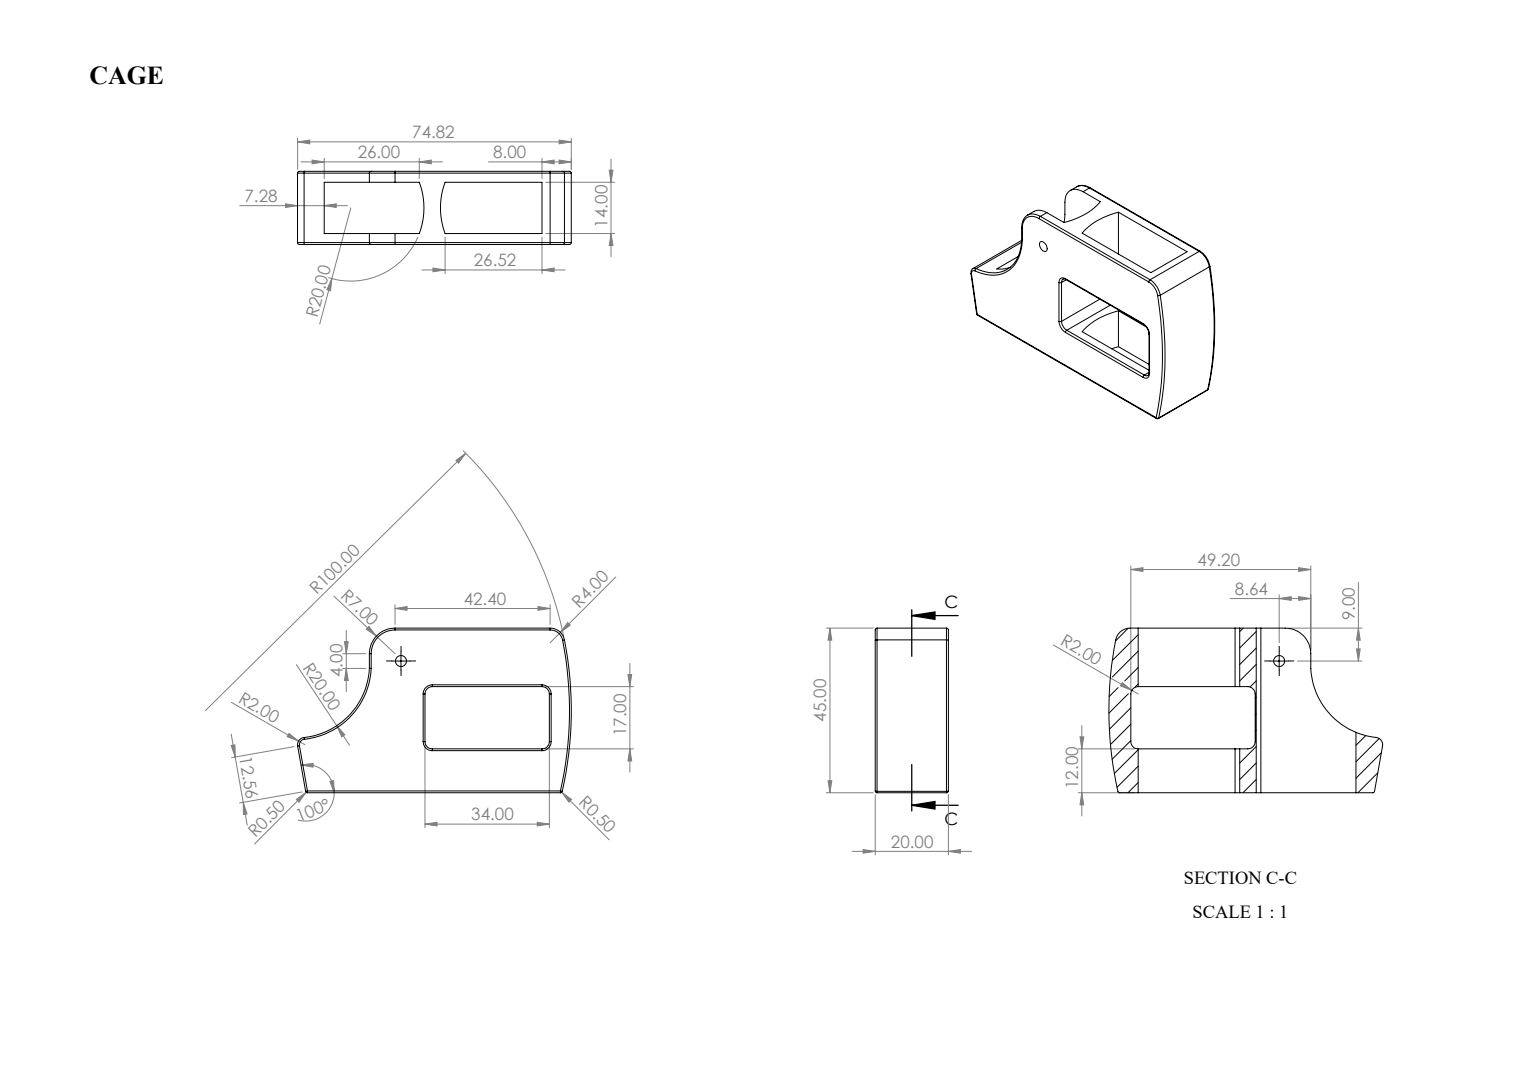
ISO-10303-21;
HEADER;
FILE_DESCRIPTION (('STEP AP214'),
    '1' );
FILE_NAME ('1.1 Cage.step',
    '2026-10-07T05:30:18',
    ( '' ),
    ( '' ),
    'SwSTEP 2.0',
    'SolidWorks 2021',
    '' );
FILE_SCHEMA (( 'AUTOMOTIVE_DESIGN' ));
ENDSEC;

DATA;
#41=DIRECTION ( 'NONE',  ( 1.000000000000000000, -5.818595309480553908E-17, 0.000000000000000000 ) ) ;
#61=ORIENTED_EDGE ( 'NONE', *, *, #8376, .F. ) ;
#102=DIRECTION ( 'NONE',  ( 0.000000000000000000, 0.000000000000000000, 1.000000000000000000 ) ) ;
#168=EDGE_LOOP ( 'NONE', ( #11039, #37677, #32498, #88509 ) ) ;
#188=DIRECTION ( 'NONE',  ( 0.000000000000000000, 0.000000000000000000, -1.000000000000000000 ) ) ;
#215=VECTOR ( 'NONE', #1501, 1000.000000000000000 ) ;
#223=DIRECTION ( 'NONE',  ( -1.000000000000000000, 0.000000000000000000, 0.000000000000000000 ) ) ;
#244=CARTESIAN_POINT ( 'NONE',  ( 17.35999999999999943, 37.99999999999997868, -7.000000000000000888 ) ) ;
#295=VERTEX_POINT ( 'NONE', #12397 ) ;
#330=ORIENTED_EDGE ( 'NONE', *, *, #68148, .F. ) ;
#338=ADVANCED_FACE ( 'NONE', ( #83350 ), #59848, .T. ) ;
#341=ORIENTED_EDGE ( 'NONE', *, *, #63443, .F. ) ;
#348=EDGE_CURVE ( 'NONE', #78868, #92229, #98382, .T. ) ;
#354=CYLINDRICAL_SURFACE ( 'NONE', #94314, 1.500000000000001332 ) ;
#363=( NAMED_UNIT ( * ) PLANE_ANGLE_UNIT ( ) SI_UNIT ( $, .RADIAN. ) );
#376=DIRECTION ( 'NONE',  ( 8.673617379884028570E-16, 1.000000000000000000, 0.000000000000000000 ) ) ;
#416=EDGE_CURVE ( 'NONE', #77981, #78868, #23450, .T. ) ;
#435=CIRCLE ( 'NONE', #56286, 0.5000000000000004441 ) ;
#442=VECTOR ( 'NONE', #21341, 1000.000000000000000 ) ;
#515=AXIS2_PLACEMENT_3D ( 'NONE', #48897, #3417, #2454 ) ;
#622=ORIENTED_EDGE ( 'NONE', *, *, #68148, .T. ) ;
#624=EDGE_CURVE ( 'NONE', #55254, #84180, #16333, .T. ) ;
#646=CIRCLE ( 'NONE', #50126, 0.5000000000000004441 ) ;
#683=EDGE_LOOP ( 'NONE', ( #89286, #70772, #2079, #80343 ) ) ;
#743=DIRECTION ( 'NONE',  ( 0.000000000000000000, 1.000000000000000000, 0.000000000000000000 ) ) ;
#779=ORIENTED_EDGE ( 'NONE', *, *, #18509, .T. ) ;
#805=ORIENTED_EDGE ( 'NONE', *, *, #45534, .F. ) ;
#821=DIRECTION ( 'NONE',  ( 1.000000000000000000, 0.000000000000000000, 5.329070518200751394E-15 ) ) ;
#842=PRODUCT_DEFINITION_FORMATION_WITH_SPECIFIED_SOURCE ( 'ANY', '', #6128, .NOT_KNOWN. ) ;
#860=DIRECTION ( 'NONE',  ( -1.000000000000000000, 0.000000000000000000, 0.000000000000000000 ) ) ;
#985=CARTESIAN_POINT ( 'NONE',  ( 32.06412365047463453, 14.00000000000001066, 9.500000000000000000 ) ) ;
#1075=VECTOR ( 'NONE', #35109, 1000.000000000000000 ) ;
#1105=LINE ( 'NONE', #77561, #75163 ) ;
#1127=DIRECTION ( 'NONE',  ( -0.000000000000000000, -0.000000000000000000, -1.000000000000000000 ) ) ;
#1194=VERTEX_POINT ( 'NONE', #53106 ) ;
#1221=CIRCLE ( 'NONE', #85851, 2.500000000000002220 ) ;
#1239=DIRECTION ( 'NONE',  ( -1.000000000000000000, 0.000000000000000000, -0.000000000000000000 ) ) ;
#1268=EDGE_CURVE ( 'NONE', #62689, #78249, #21639, .T. ) ;
#1292=ORIENTED_EDGE ( 'NONE', *, *, #36512, .F. ) ;
#1301=AXIS2_PLACEMENT_3D ( 'NONE', #24699, #5022, #40184 ) ;
#1353=CARTESIAN_POINT ( 'NONE',  ( 56.78206182523731371, 11.99999999999999645, 0.000000000000000000 ) ) ;
#1361=DIRECTION ( 'NONE',  ( -1.000000000000000000, 0.000000000000000000, 0.000000000000000000 ) ) ;
#1429=AXIS2_PLACEMENT_3D ( 'NONE', #13943, #37436, #81435 ) ;
#1435=EDGE_LOOP ( 'NONE', ( #67910, #41636, #41848, #61382 ) ) ;
#1462=CARTESIAN_POINT ( 'NONE',  ( 34.56412365047464874, 28.99999999999999645, -9.500000000000000000 ) ) ;
#1501=DIRECTION ( 'NONE',  ( -5.818595309480553908E-17, -1.000000000000000000, -0.000000000000000000 ) ) ;
#1530=ORIENTED_EDGE ( 'NONE', *, *, #39660, .F. ) ;
#1573=ORIENTED_EDGE ( 'NONE', *, *, #56390, .F. ) ;
#1574=CARTESIAN_POINT ( 'NONE',  ( 66.76470751278411342, 44.49999999999998579, -10.00000000000000000 ) ) ;
#1577=AXIS2_PLACEMENT_3D ( 'NONE', #56614, #86134, #18135 ) ;
#1599=ADVANCED_FACE ( 'NONE', ( #9580 ), #1613, .T. ) ;
#1613=CYLINDRICAL_SURFACE ( 'NONE', #68754, 0.5000000000000000000 ) ;
#1615=EDGE_CURVE ( 'NONE', #75199, #35183, #12837, .T. ) ;
#1641=EDGE_LOOP ( 'NONE', ( #14568, #34746, #43556, #39557 ) ) ;
#1655=ADVANCED_FACE ( 'NONE', ( #38607 ), #78570, .T. ) ;
#1722=EDGE_CURVE ( 'NONE', #68545, #40747, #20847, .T. ) ;
#1775=LINE ( 'NONE', #9251, #65321 ) ;
#1777=DIRECTION ( 'NONE',  ( 1.000000000000000000, -5.818595309480552676E-17, 0.000000000000000000 ) ) ;
#1778=VERTEX_POINT ( 'NONE', #71570 ) ;
#1806=DIRECTION ( 'NONE',  ( 1.000000000000000000, 0.000000000000000000, 0.000000000000000000 ) ) ;
#1830=VECTOR ( 'NONE', #23097, 1000.000000000000000 ) ;
#1855=EDGE_CURVE ( 'NONE', #77981, #81201, #86570, .T. ) ;
#1891=EDGE_CURVE ( 'NONE', #46560, #16030, #51044, .T. ) ;
#1923=DIRECTION ( 'NONE',  ( 1.000000000000000000, 0.000000000000000000, 0.000000000000000000 ) ) ;
#2052=ORIENTED_EDGE ( 'NONE', *, *, #45045, .T. ) ;
#2071=VECTOR ( 'NONE', #29687, 1000.000000000000000 ) ;
#2079=ORIENTED_EDGE ( 'NONE', *, *, #57225, .T. ) ;
#2148=CIRCLE ( 'NONE', #34070, 2.000000000000001776 ) ;
#2156=DIRECTION ( 'NONE',  ( -1.000000000000000000, 0.000000000000000000, 0.000000000000000000 ) ) ;
#2318=DIRECTION ( 'NONE',  ( -0.000000000000000000, -0.000000000000000000, -1.000000000000000000 ) ) ;
#2410=DIRECTION ( 'NONE',  ( -0.000000000000000000, -0.000000000000000000, 1.000000000000000000 ) ) ;
#2441=VECTOR ( 'NONE', #86202, 1000.000000000000000 ) ;
#2454=DIRECTION ( 'NONE',  ( -1.000000000000000000, 0.000000000000000000, 0.000000000000000000 ) ) ;
#2463=DIRECTION ( 'NONE',  ( -1.000000000000000000, 0.000000000000000000, 0.000000000000000000 ) ) ;
#2601=CARTESIAN_POINT ( 'NONE',  ( 64.56412365047461321, 11.49999999999999289, -9.500000000000000000 ) ) ;
#2602=VECTOR ( 'NONE', #71219, 1000.000000000000000 ) ;
#2603=VECTOR ( 'NONE', #71659, 1000.000000000000000 ) ;
#2681=LINE ( 'NONE', #40163, #5977 ) ;
#2687=CARTESIAN_POINT ( 'NONE',  ( 69.60148758828984228, 0.4999999999999982792, -9.500000000000000000 ) ) ;
#2732=EDGE_LOOP ( 'NONE', ( #59068, #59314, #36568, #45789 ) ) ;
#2744=FACE_OUTER_BOUND ( 'NONE', #54008, .T. ) ;
#2757=ADVANCED_FACE ( 'NONE', ( #13268 ), #12772, .T. ) ;
#2765=ORIENTED_EDGE ( 'NONE', *, *, #69274, .F. ) ;
#2825=CARTESIAN_POINT ( 'NONE',  ( 64.56412365047461321, 11.99999999999999467, 9.500000000000000000 ) ) ;
#2884=ORIENTED_EDGE ( 'NONE', *, *, #5462, .T. ) ;
#2912=CARTESIAN_POINT ( 'NONE',  ( -2.614810775378867191, 35.00346125376525919, -9.500000000000000000 ) ) ;
#3082=DIRECTION ( 'NONE',  ( -1.000000000000000000, 0.000000000000000000, 0.000000000000000000 ) ) ;
#3176=FACE_OUTER_BOUND ( 'NONE', #51806, .T. ) ;
#3186=CARTESIAN_POINT ( 'NONE',  ( 34.56412365047463453, 26.99999999999999645, 9.500000000000000000 ) ) ;
#3235=ORIENTED_EDGE ( 'NONE', *, *, #67059, .F. ) ;
#3239=ORIENTED_EDGE ( 'NONE', *, *, #59709, .T. ) ;
#3260=DIRECTION ( 'NONE',  ( -1.000000000000000000, 0.000000000000000000, 0.000000000000000000 ) ) ;
#3261=CARTESIAN_POINT ( 'NONE',  ( 34.56412365047464874, 11.99999999999999645, -9.500000000000000000 ) ) ;
#3266=DIRECTION ( 'NONE',  ( 0.000000000000000000, 0.000000000000000000, -1.000000000000000000 ) ) ;
#3269=CARTESIAN_POINT ( 'NONE',  ( -0.2838433074297238012, 13.12729635533385597, 10.00000000000000000 ) ) ;
#3417=DIRECTION ( 'NONE',  ( -0.000000000000000000, -0.000000000000000000, -1.000000000000000000 ) ) ;
#3456=AXIS2_PLACEMENT_3D ( 'NONE', #58748, #73747, #74740 ) ;
#3466=ORIENTED_EDGE ( 'NONE', *, *, #7847, .T. ) ;
#3528=ORIENTED_EDGE ( 'NONE', *, *, #92910, .F. ) ;
#3546=VERTEX_POINT ( 'NONE', #61597 ) ;
#3627=AXIS2_PLACEMENT_3D ( 'NONE', #11825, #31981, #54984 ) ;
#3661=CARTESIAN_POINT ( 'NONE',  ( 24.35999999999999233, 44.99999999999997158, -9.500000000000000000 ) ) ;
#3664=ORIENTED_EDGE ( 'NONE', *, *, #18435, .F. ) ;
#3673=DIRECTION ( 'NONE',  ( -0.000000000000000000, -0.000000000000000000, -1.000000000000000000 ) ) ;
#3728=DIRECTION ( 'NONE',  ( 0.000000000000000000, 0.000000000000000000, 1.000000000000000000 ) ) ;
#3741=EDGE_CURVE ( 'NONE', #63150, #37315, #33075, .T. ) ;
#3766=EDGE_CURVE ( 'NONE', #44163, #68545, #38622, .T. ) ;
#3904=VECTOR ( 'NONE', #60597, 1000.000000000000000 ) ;
#3910=DIRECTION ( 'NONE',  ( 0.000000000000000000, -1.000000000000000000, 0.000000000000000000 ) ) ;
#3952=LINE ( 'NONE', #71474, #73349 ) ;
#3998=ADVANCED_FACE ( 'NONE', ( #51481, #13487 ), #74469, .T. ) ;
#4006=VERTEX_POINT ( 'NONE', #54428 ) ;
#4062=CARTESIAN_POINT ( 'NONE',  ( 24.35999999999999233, 37.99999999999997868, -9.500000000000000000 ) ) ;
#4069=CARTESIAN_POINT ( 'NONE',  ( -27.43587634952538323, 44.49999999999997158, 9.500000000000000000 ) ) ;
#4131=VECTOR ( 'NONE', #74732, 1000.000000000000000 ) ;
#4133=ORIENTED_EDGE ( 'NONE', *, *, #15488, .F. ) ;
#4150=LINE ( 'NONE', #65111, #1075 ) ;
#4170=EDGE_CURVE ( 'NONE', #3546, #61160, #15953, .T. ) ;
#4210=DIRECTION ( 'NONE',  ( 0.000000000000000000, 0.000000000000000000, -1.000000000000000000 ) ) ;
#4243=LINE ( 'NONE', #27213, #33587 ) ;
#4245=EDGE_CURVE ( 'NONE', #48019, #20819, #7882, .T. ) ;
#4282=DIRECTION ( 'NONE',  ( -0.000000000000000000, -0.000000000000000000, 1.000000000000000000 ) ) ;
#4296=DIRECTION ( 'NONE',  ( 1.000000000000000000, -5.818595309480553908E-17, 0.000000000000000000 ) ) ;
#4299=LINE ( 'NONE', #34773, #71110 ) ;
#4386=DIRECTION ( 'NONE',  ( 1.000000000000000000, -5.818595309480553908E-17, 0.000000000000000000 ) ) ;
#4391=ORIENTED_EDGE ( 'NONE', *, *, #11802, .T. ) ;
#4442=CARTESIAN_POINT ( 'NONE',  ( 24.35999999999999233, 44.99999999999997868, 9.500000000000000000 ) ) ;
#4446=EDGE_CURVE ( 'NONE', #35322, #77981, #80390, .T. ) ;
#4506=DIRECTION ( 'NONE',  ( 0.000000000000000000, 0.000000000000000000, -1.000000000000000000 ) ) ;
#4534=VECTOR ( 'NONE', #5458, 1000.000000000000000 ) ;
#4611=ORIENTED_EDGE ( 'NONE', *, *, #67459, .T. ) ;
#4631=EDGE_CURVE ( 'NONE', #49611, #61145, #13868, .T. ) ;
#4639=ORIENTED_EDGE ( 'NONE', *, *, #37254, .F. ) ;
#4650=CARTESIAN_POINT ( 'NONE',  ( -2.253458813454140675, 12.77999999999999936, 10.00000000000000000 ) ) ;
#4673=CARTESIAN_POINT ( 'NONE',  ( -1.783843307429720415, 13.12729635533385597, 9.500000000000000000 ) ) ;
#4764=EDGE_CURVE ( 'NONE', #82054, #63150, #83025, .T. ) ;
#4873=CARTESIAN_POINT ( 'NONE',  ( 2.618367889266248100E-15, 44.99999999999999289, -7.000000000000000000 ) ) ;
#4901=DIRECTION ( 'NONE',  ( 0.000000000000000000, 1.000000000000000000, 0.000000000000000000 ) ) ;
#4904=ADVANCED_FACE ( 'NONE', ( #29341 ), #14366, .T. ) ;
#4907=FACE_OUTER_BOUND ( 'NONE', #90936, .T. ) ;
#4935=ORIENTED_EDGE ( 'NONE', *, *, #41909, .F. ) ;
#4969=VECTOR ( 'NONE', #81230, 1000.000000000000000 ) ;
#5022=DIRECTION ( 'NONE',  ( -0.000000000000000000, -0.000000000000000000, -1.000000000000000000 ) ) ;
#5073=LINE ( 'NONE', #35052, #35515 ) ;
#5124=DIRECTION ( 'NONE',  ( -1.000000000000000000, 5.818595309480552676E-17, 0.000000000000000000 ) ) ;
#5133=ORIENTED_EDGE ( 'NONE', *, *, #57378, .T. ) ;
#5280=ADVANCED_FACE ( 'NONE', ( #45224 ), #78296, .T. ) ;
#5288=CARTESIAN_POINT ( 'NONE',  ( 24.35999999999999233, 44.49999999999997868, 10.00000000000000000 ) ) ;
#5307=TOROIDAL_SURFACE ( 'NONE', #89936, 2.500000000000001776, 0.5000000000000000000 ) ;
#5354=ORIENTED_EDGE ( 'NONE', *, *, #28574, .F. ) ;
#5376=ADVANCED_FACE ( 'NONE', ( #30209 ), #75994, .T. ) ;
#5407=DIRECTION ( 'NONE',  ( 0.000000000000000000, 1.000000000000000000, 0.000000000000000000 ) ) ;
#5431=EDGE_CURVE ( 'NONE', #15047, #60197, #18477, .T. ) ;
#5458=DIRECTION ( 'NONE',  ( -0.000000000000000000, 1.000000000000000000, -0.000000000000000000 ) ) ;
#5462=EDGE_CURVE ( 'NONE', #49611, #11195, #38233, .T. ) ;
#5674=ORIENTED_EDGE ( 'NONE', *, *, #84120, .T. ) ;
#5727=DIRECTION ( 'NONE',  ( 1.000000000000000000, 0.000000000000000000, 0.000000000000000000 ) ) ;
#5730=CYLINDRICAL_SURFACE ( 'NONE', #81897, 0.5000000000000004441 ) ;
#5792=CIRCLE ( 'NONE', #21789, 6.999999999999995559 ) ;
#5882=DIRECTION ( 'NONE',  ( 1.000000000000000000, 1.636349903325072848E-16, 0.000000000000000000 ) ) ;
#5907=CARTESIAN_POINT ( 'NONE',  ( 32.56412365047463453, 26.99999999999998224, 10.00000000000000000 ) ) ;
#5977=VECTOR ( 'NONE', #25179, 1000.000000000000000 ) ;
#5988=CARTESIAN_POINT ( 'NONE',  ( 24.50000000000000000, 35.99999999999997158, -10.00000000000000000 ) ) ;
#6010=ORIENTED_EDGE ( 'NONE', *, *, #68078, .T. ) ;
#6013=AXIS2_PLACEMENT_3D ( 'NONE', #63863, #34354, #33853 ) ;
#6038=VERTEX_POINT ( 'NONE', #81127 ) ;
#6041=ADVANCED_FACE ( 'NONE', ( #43128 ), #98366, .T. ) ;
#6085=ORIENTED_EDGE ( 'NONE', *, *, #65380, .F. ) ;
#6128=PRODUCT ( '1.1 Cage', '1.1 Cage', '', ( #23222 ) ) ;
#6137=DIRECTION ( 'NONE',  ( 0.000000000000000000, -1.000000000000000000, 0.000000000000000000 ) ) ;
#6193=CARTESIAN_POINT ( 'NONE',  ( 24.35999999999999233, 37.99999999999997868, -10.00000000000000000 ) ) ;
#6273=DIRECTION ( 'NONE',  ( -5.818595309480553908E-17, -1.000000000000000000, -0.000000000000000000 ) ) ;
#6290=LINE ( 'NONE', #67287, #48607 ) ;
#6310=ORIENTED_EDGE ( 'NONE', *, *, #31051, .T. ) ;
#6358=ORIENTED_EDGE ( 'NONE', *, *, #24550, .F. ) ;
#6408=AXIS2_PLACEMENT_3D ( 'NONE', #52884, #30143, #188 ) ;
#6535=AXIS2_PLACEMENT_3D ( 'NONE', #7124, #53598, #90608 ) ;
#6556=VERTEX_POINT ( 'NONE', #93438 ) ;
#6603=AXIS2_PLACEMENT_3D ( 'NONE', #4673, #6137, #27144 ) ;
#6623=CARTESIAN_POINT ( 'NONE',  ( 70.00000000000000000, -4.073016716636387686E-15, 9.500000000000000000 ) ) ;
#6624=DIRECTION ( 'NONE',  ( -0.1736481776669272503, 0.9848077530122086864, -0.000000000000000000 ) ) ;
#6701=FACE_OUTER_BOUND ( 'NONE', #42927, .T. ) ;
#6709=ORIENTED_EDGE ( 'NONE', *, *, #20199, .T. ) ;
#6723=SHAPE_DEFINITION_REPRESENTATION ( #13299, #53719 ) ;
#6789=CARTESIAN_POINT ( 'NONE',  ( 17.35999999999999943, 33.99999999999997158, 9.500000000000000000 ) ) ;
#6855=CARTESIAN_POINT ( 'NONE',  ( -27.43587634952537968, 29.50000000000000000, -9.500000000000000000 ) ) ;
#6862=DIRECTION ( 'NONE',  ( 0.000000000000000000, 0.000000000000000000, 1.000000000000000000 ) ) ;
#7000=DIRECTION ( 'NONE',  ( -1.000000000000000000, 0.000000000000000000, 0.000000000000000000 ) ) ;
#7017=EDGE_CURVE ( 'NONE', #12064, #61160, #19891, .T. ) ;
#7040=ORIENTED_EDGE ( 'NONE', *, *, #44146, .F. ) ;
#7056=CIRCLE ( 'NONE', #59697, 2.500000000000002220 ) ;
#7124=CARTESIAN_POINT ( 'NONE',  ( 64.56412365047462742, 13.99999999999999467, -10.00000000000000000 ) ) ;
#7201=CARTESIAN_POINT ( 'NONE',  ( 2.618367889266248100E-15, 44.99999999999999289, 7.000000000000000000 ) ) ;
#7217=DIRECTION ( 'NONE',  ( 0.000000000000000000, 0.000000000000000000, 1.000000000000000000 ) ) ;
#7257=CARTESIAN_POINT ( 'NONE',  ( 34.56412365047463453, 13.99999999999999645, -9.500000000000000000 ) ) ;
#7301=ORIENTED_EDGE ( 'NONE', *, *, #57955, .T. ) ;
#7332=DIRECTION ( 'NONE',  ( 1.000000000000000000, 0.000000000000000000, 0.000000000000000000 ) ) ;
#7426=ORIENTED_EDGE ( 'NONE', *, *, #54855, .T. ) ;
#7448=MECHANICAL_DESIGN_GEOMETRIC_PRESENTATION_REPRESENTATION('',(#55310),#40777);
#7451=ORIENTED_EDGE ( 'NONE', *, *, #10767, .F. ) ;
#7470=ORIENTED_EDGE ( 'NONE', *, *, #63443, .T. ) ;
#7496=AXIS2_PLACEMENT_3D ( 'NONE', #84136, #7656, #70606 ) ;
#7500=VECTOR ( 'NONE', #33517, 1000.000000000000000 ) ;
#7501=ADVANCED_FACE ( 'NONE', ( #65258 ), #63136, .T. ) ;
#7502=ORIENTED_EDGE ( 'NONE', *, *, #89283, .F. ) ;
#7529=CARTESIAN_POINT ( 'NONE',  ( 17.85999999999999943, 37.99999999999997868, 9.500000000000000000 ) ) ;
#7636=CIRCLE ( 'NONE', #92271, 99.50000000000000000 ) ;
#7656=DIRECTION ( 'NONE',  ( 1.000000000000000000, 0.000000000000000000, 0.000000000000000000 ) ) ;
#7710=EDGE_CURVE ( 'NONE', #62689, #39764, #83849, .T. ) ;
#7735=EDGE_CURVE ( 'NONE', #35951, #20172, #91847, .T. ) ;
#7793=ORIENTED_EDGE ( 'NONE', *, *, #4245, .T. ) ;
#7805=EDGE_LOOP ( 'NONE', ( #30049, #60359, #7502, #60391 ) ) ;
#7847=EDGE_CURVE ( 'NONE', #35983, #13186, #18198, .T. ) ;
#7853=DIRECTION ( 'NONE',  ( -0.000000000000000000, -0.000000000000000000, -1.000000000000000000 ) ) ;
#7857=CARTESIAN_POINT ( 'NONE',  ( 2.241241388159942801E-47, 3.851859888774471706E-31, 7.000000000000000000 ) ) ;
#7882=CIRCLE ( 'NONE', #63734, 19.99999999999999289 ) ;
#7993=CARTESIAN_POINT ( 'NONE',  ( 5.000000000000002665, 44.99999999999999289, -7.000000000000000000 ) ) ;
#8024=CARTESIAN_POINT ( 'NONE',  ( 64.56412365047462742, 26.99999999999999645, -9.500000000000000000 ) ) ;
#8175=EDGE_CURVE ( 'NONE', #75802, #25854, #25049, .T. ) ;
#8223=DIRECTION ( 'NONE',  ( -1.000000000000000000, 0.000000000000000000, 0.000000000000000000 ) ) ;
#8280=EDGE_CURVE ( 'NONE', #62619, #94846, #34972, .T. ) ;
#8308=CARTESIAN_POINT ( 'NONE',  ( 56.78206182523731371, 44.99999999999999289, 0.000000000000000000 ) ) ;
#8343=DIRECTION ( 'NONE',  ( 0.000000000000000000, 0.000000000000000000, 1.000000000000000000 ) ) ;
#8376=EDGE_CURVE ( 'NONE', #13186, #50694, #35965, .T. ) ;
#8489=LINE ( 'NONE', #68996, #72048 ) ;
#8493=EDGE_CURVE ( 'NONE', #75199, #87279, #49875, .T. ) ;
#8513=ORIENTED_EDGE ( 'NONE', *, *, #44034, .T. ) ;
#8533=ORIENTED_EDGE ( 'NONE', *, *, #48100, .F. ) ;
#8605=ADVANCED_FACE ( 'NONE', ( #37468 ), #61420, .F. ) ;
#8624=EDGE_LOOP ( 'NONE', ( #77958, #17574, #54506, #22214 ) ) ;
#8666=DIRECTION ( 'NONE',  ( -1.000000000000000000, 0.000000000000000000, 0.000000000000000000 ) ) ;
#8678=CARTESIAN_POINT ( 'NONE',  ( 17.35999999999999588, 33.99999999999997158, 7.000000000000000000 ) ) ;
#8903=EDGE_CURVE ( 'NONE', #69260, #50813, #83447, .T. ) ;
#8918=DIRECTION ( 'NONE',  ( -1.000000000000000000, 3.538835890992686473E-15, 0.000000000000000000 ) ) ;
#8927=ADVANCED_FACE ( 'NONE', ( #45947 ), #30921, .T. ) ;
#9111=AXIS2_PLACEMENT_3D ( 'NONE', #63896, #49887, #94409 ) ;
#9193=DIRECTION ( 'NONE',  ( 0.1059530667249611452, -0.9943711317468825195, 0.000000000000000000 ) ) ;
#9251=CARTESIAN_POINT ( 'NONE',  ( 17.85999999999999943, 37.99999999999997868, -10.00000000000000000 ) ) ;
#9261=EDGE_CURVE ( 'NONE', #40893, #89049, #94630, .T. ) ;
#9273=DIRECTION ( 'NONE',  ( -1.000000000000000000, -1.636349903325072848E-16, 0.000000000000000000 ) ) ;
#9274=CARTESIAN_POINT ( 'NONE',  ( 2.241241388159942801E-47, 3.851859888774471706E-31, -7.000000000000000000 ) ) ;
#9322=CARTESIAN_POINT ( 'NONE',  ( 2.618367889266248100E-15, 44.99999999999999289, 7.000000000000000000 ) ) ;
#9366=ORIENTED_EDGE ( 'NONE', *, *, #58135, .F. ) ;
#9369=ORIENTED_EDGE ( 'NONE', *, *, #54989, .T. ) ;
#9390=CARTESIAN_POINT ( 'NONE',  ( 26.00000000000000355, 35.99999999999997158, -10.00000000000000000 ) ) ;
#9432=DIRECTION ( 'NONE',  ( 1.000000000000000000, -5.818595309480553908E-17, 0.000000000000000000 ) ) ;
#9443=CARTESIAN_POINT ( 'NONE',  ( 24.50000000000000000, 35.99999999999997158, -10.00000000000000000 ) ) ;
#9458=CARTESIAN_POINT ( 'NONE',  ( 64.56412365047461321, -3.756725070333740926E-15, 7.000000000000000000 ) ) ;
#9580=FACE_OUTER_BOUND ( 'NONE', #2732, .T. ) ;
#9602=DIRECTION ( 'NONE',  ( -0.000000000000000000, -0.000000000000000000, -1.000000000000000000 ) ) ;
#9689=DIRECTION ( 'NONE',  ( -1.000000000000000000, 0.000000000000000000, 0.000000000000000000 ) ) ;
#9709=DIRECTION ( 'NONE',  ( -1.000000000000000000, 0.000000000000000000, 0.000000000000000000 ) ) ;
#9723=CARTESIAN_POINT ( 'NONE',  ( -0.07285406091746288171, 0.4131759111665359585, 10.00000000000000000 ) ) ;
#9724=AXIS2_PLACEMENT_3D ( 'NONE', #48543, #56547, #87042 ) ;
#9991=ORIENTED_EDGE ( 'NONE', *, *, #54745, .F. ) ;
#10044=CIRCLE ( 'NONE', #96262, 1.500000000000001332 ) ;
#10079=CARTESIAN_POINT ( 'NONE',  ( 17.85999999999998522, 22.49999999999995026, 9.500000000000000000 ) ) ;
#10130=ORIENTED_EDGE ( 'NONE', *, *, #59434, .F. ) ;
#10146=ORIENTED_EDGE ( 'NONE', *, *, #63448, .F. ) ;
#10249=ORIENTED_EDGE ( 'NONE', *, *, #3741, .T. ) ;
#10274=DIRECTION ( 'NONE',  ( 0.000000000000000000, 1.000000000000000000, 0.000000000000000000 ) ) ;
#10313=ORIENTED_EDGE ( 'NONE', *, *, #28574, .T. ) ;
#10338=CARTESIAN_POINT ( 'NONE',  ( 24.35999999999999233, 44.49999999999997868, -10.00000000000000000 ) ) ;
#10519=AXIS2_PLACEMENT_3D ( 'NONE', #25436, #77413, #69937 ) ;
#10652=DIRECTION ( 'NONE',  ( 1.000000000000000000, 0.000000000000000000, 0.000000000000000000 ) ) ;
#10657=AXIS2_PLACEMENT_3D ( 'NONE', #76337, #7853, #75845 ) ;
#10761=EDGE_CURVE ( 'NONE', #15070, #66451, #24301, .T. ) ;
#10763=CARTESIAN_POINT ( 'NONE',  ( 31.00000000000000000, -1.803315223424012063E-15, -7.000000000000000000 ) ) ;
#10767=EDGE_CURVE ( 'NONE', #44163, #42904, #55111, .T. ) ;
#10785=VERTEX_POINT ( 'NONE', #62764 ) ;
#10816=VERTEX_POINT ( 'NONE', #46779 ) ;
#10833=CIRCLE ( 'NONE', #49144, 0.4999999999999995559 ) ;
#10853=DIRECTION ( 'NONE',  ( -0.000000000000000000, -0.000000000000000000, -1.000000000000000000 ) ) ;
#10878=ORIENTED_EDGE ( 'NONE', *, *, #3741, .F. ) ;
#10939=CARTESIAN_POINT ( 'NONE',  ( -1.783843307429720415, 13.12729635533385597, 10.00000000000000000 ) ) ;
#10978=EDGE_CURVE ( 'NONE', #25147, #92057, #87393, .T. ) ;
#11039=ORIENTED_EDGE ( 'NONE', *, *, #68784, .F. ) ;
#11122=FILL_AREA_STYLE_COLOUR ( '', #98464 ) ;
#11131=CARTESIAN_POINT ( 'NONE',  ( 4.999999999999997335, 16.50982297312470592, 7.000000000000000000 ) ) ;
#11139=DIRECTION ( 'NONE',  ( 0.000000000000000000, 1.000000000000000000, 0.000000000000000000 ) ) ;
#11192=CIRCLE ( 'NONE', #92633, 2.000000000000001776 ) ;
#11195=VERTEX_POINT ( 'NONE', #30055 ) ;
#11231=VERTEX_POINT ( 'NONE', #89583 ) ;
#11238=EDGE_CURVE ( 'NONE', #25147, #12064, #15557, .T. ) ;
#11313=TOROIDAL_SURFACE ( 'NONE', #71981, 99.50000000000000000, 0.5000000000000000000 ) ;
#11334=VERTEX_POINT ( 'NONE', #30548 ) ;
#11336=EDGE_LOOP ( 'NONE', ( #55541, #47242, #44700, #68412 ) ) ;
#11403=CARTESIAN_POINT ( 'NONE',  ( 17.72850354356589619, 33.99078749795493337, -9.999999999999998224 ) ) ;
#11406=EDGE_LOOP ( 'NONE', ( #51286, #83677, #74403, #25901, #5133, #59629, #49323, #43801, #43659, #33434 ) ) ;
#11417=ORIENTED_EDGE ( 'NONE', *, *, #62641, .T. ) ;
#11498=EDGE_LOOP ( 'NONE', ( #71210, #1573, #92198 ) ) ;
#11499=CIRCLE ( 'NONE', #37075, 0.4999999999999998335 ) ;
#11521=AXIS2_PLACEMENT_3D ( 'NONE', #35206, #41760, #3260 ) ;
#11609=SURFACE_STYLE_FILL_AREA ( #50598 ) ;
#11630=FACE_OUTER_BOUND ( 'NONE', #8624, .T. ) ;
#11650=CARTESIAN_POINT ( 'NONE',  ( 64.56412365047461321, 44.99999999999998579, 7.000000000000000000 ) ) ;
#11794=LINE ( 'NONE', #98661, #71855 ) ;
#11802=EDGE_CURVE ( 'NONE', #51757, #39764, #48228, .T. ) ;
#11806=AXIS2_PLACEMENT_3D ( 'NONE', #17734, #61729, #54236 ) ;
#11825=CARTESIAN_POINT ( 'NONE',  ( 2.618367889266248100E-15, 44.99999999999999289, 7.000000000000000000 ) ) ;
#11919=DIRECTION ( 'NONE',  ( 0.000000000000000000, 0.000000000000000000, 1.000000000000000000 ) ) ;
#11948=DIRECTION ( 'NONE',  ( 1.000000000000000000, -5.818595309480552676E-17, -0.000000000000000000 ) ) ;
#12064=VERTEX_POINT ( 'NONE', #26224 ) ;
#12131=DIRECTION ( 'NONE',  ( 0.000000000000000000, 0.000000000000000000, 1.000000000000000000 ) ) ;
#12138=DIRECTION ( 'NONE',  ( -1.000000000000000000, 0.000000000000000000, 0.000000000000000000 ) ) ;
#12185=CARTESIAN_POINT ( 'NONE',  ( -1.783843307429720415, 13.12729635533385597, -9.500000000000000000 ) ) ;
#12397=CARTESIAN_POINT ( 'NONE',  ( 64.56412365047461321, 11.99999999999999467, 9.500000000000000000 ) ) ;
#12604=DIRECTION ( 'NONE',  ( 1.000000000000000000, 6.938893903907222067E-15, 0.000000000000000000 ) ) ;
#12611=DIRECTION ( 'NONE',  ( -0.000000000000000000, -0.000000000000000000, -1.000000000000000000 ) ) ;
#12640=CARTESIAN_POINT ( 'NONE',  ( 26.00000000000000355, 35.99999999999997158, -10.00000000000000000 ) ) ;
#12663=DIRECTION ( 'NONE',  ( 0.000000000000000000, 0.000000000000000000, 1.000000000000000000 ) ) ;
#12686=EDGE_CURVE ( 'NONE', #35060, #37315, #58697, .T. ) ;
#12687=AXIS2_PLACEMENT_3D ( 'NONE', #65689, #95715, #42710 ) ;
#12728=DIRECTION ( 'NONE',  ( -0.000000000000000000, -0.000000000000000000, -1.000000000000000000 ) ) ;
#12772=CYLINDRICAL_SURFACE ( 'NONE', #17296, 0.5000000000000004441 ) ;
#12809=ORIENTED_EDGE ( 'NONE', *, *, #8175, .F. ) ;
#12837=CIRCLE ( 'NONE', #81504, 4.000000000000003553 ) ;
#12957=AXIS2_PLACEMENT_3D ( 'NONE', #7529, #97547, #52996 ) ;
#12972=ORIENTED_EDGE ( 'NONE', *, *, #27212, .F. ) ;
#13000=ORIENTED_EDGE ( 'NONE', *, *, #4764, .T. ) ;
#13006=CARTESIAN_POINT ( 'NONE',  ( 66.56412365047464164, 26.99999999999998224, 9.500000000000000000 ) ) ;
#13039=EDGE_CURVE ( 'NONE', #29252, #23929, #23424, .T. ) ;
#13139=CARTESIAN_POINT ( 'NONE',  ( 5.000000000000000000, -2.909297654740273256E-16, 7.000000000000000000 ) ) ;
#13182=ORIENTED_EDGE ( 'NONE', *, *, #8175, .T. ) ;
#13186=VERTEX_POINT ( 'NONE', #8678 ) ;
#13268=FACE_OUTER_BOUND ( 'NONE', #29218, .T. ) ;
#13299=PRODUCT_DEFINITION_SHAPE ( 'NONE', 'NONE',  #66632 ) ;
#13331=ORIENTED_EDGE ( 'NONE', *, *, #78782, .T. ) ;
#13451=ORIENTED_EDGE ( 'NONE', *, *, #92279, .T. ) ;
#13461=FACE_OUTER_BOUND ( 'NONE', #26684, .T. ) ;
#13487=FACE_OUTER_BOUND ( 'NONE', #25345, .T. ) ;
#13597=EDGE_CURVE ( 'NONE', #48019, #25948, #40660, .T. ) ;
#13737=CARTESIAN_POINT ( 'NONE',  ( 64.56412365047462742, 26.99999999999999645, -9.500000000000000000 ) ) ;
#13868=LINE ( 'NONE', #38837, #47884 ) ;
#13943=CARTESIAN_POINT ( 'NONE',  ( 26.00000000000000355, 35.99999999999997158, -10.00000000000000000 ) ) ;
#13966=B_SPLINE_CURVE_WITH_KNOTS ( 'NONE', 3,
 ( #47919, #11403, #78424, #64390, #49396, #32919 ),
 .UNSPECIFIED., .F., .F.,
 ( 4, 2, 4 ),
 ( -2.009308255747123417E-05, 0.0003744380149044849223, 0.0007689691123664410110 ),
 .UNSPECIFIED. ) ;
#14061=EDGE_CURVE ( 'NONE', #11195, #35060, #70056, .T. ) ;
#14070=ORIENTED_EDGE ( 'NONE', *, *, #42833, .F. ) ;
#14193=VECTOR ( 'NONE', #90653, 1000.000000000000000 ) ;
#14198=EDGE_LOOP ( 'NONE', ( #60443, #95638, #75663, #17396 ) ) ;
#14324=CARTESIAN_POINT ( 'NONE',  ( 24.50000000000000000, 35.99999999999997158, -7.000000000000000000 ) ) ;
#14366=CYLINDRICAL_SURFACE ( 'NONE', #59032, 0.5000000000000004441 ) ;
#14441=ORIENTED_EDGE ( 'NONE', *, *, #45534, .T. ) ;
#14454=ORIENTED_EDGE ( 'NONE', *, *, #1891, .F. ) ;
#14467=DIRECTION ( 'NONE',  ( 0.000000000000000000, 0.000000000000000000, 1.000000000000000000 ) ) ;
#14568=ORIENTED_EDGE ( 'NONE', *, *, #67459, .F. ) ;
#14598=EDGE_CURVE ( 'NONE', #18488, #66580, #1775, .T. ) ;
#14607=ORIENTED_EDGE ( 'NONE', *, *, #78016, .T. ) ;
#14614=CARTESIAN_POINT ( 'NONE',  ( 34.56412365047464874, 11.99999999999999645, -9.500000000000000000 ) ) ;
#14644=LINE ( 'NONE', #37138, #52990 ) ;
#14686=ORIENTED_EDGE ( 'NONE', *, *, #41019, .F. ) ;
#14689=EDGE_LOOP ( 'NONE', ( #80068, #97209, #57071, #73354 ) ) ;
#14722=DIRECTION ( 'NONE',  ( -0.000000000000000000, -0.000000000000000000, -1.000000000000000000 ) ) ;
#14775=AXIS2_PLACEMENT_3D ( 'NONE', #12185, #27180, #4210 ) ;
#14790=AXIS2_PLACEMENT_3D ( 'NONE', #83391, #14909, #45381 ) ;
#14817=ADVANCED_FACE ( 'NONE', ( #81757 ), #29255, .T. ) ;
#14820=AXIS2_PLACEMENT_3D ( 'NONE', #89938, #82437, #88959 ) ;
#14821=ORIENTED_EDGE ( 'NONE', *, *, #27965, .T. ) ;
#14839=TOROIDAL_SURFACE ( 'NONE', #515, 3.500000000000000888, 0.5000000000000000000 ) ;
#14857=FILL_AREA_STYLE ('',( #21857 ) ) ;
#14868=DIRECTION ( 'NONE',  ( -1.000000000000000000, 0.000000000000000000, 0.000000000000000000 ) ) ;
#14876=LINE ( 'NONE', #7857, #52291 ) ;
#14909=DIRECTION ( 'NONE',  ( -0.000000000000000000, -0.000000000000000000, -1.000000000000000000 ) ) ;
#14925=EDGE_CURVE ( 'NONE', #61145, #10785, #38258, .T. ) ;
#14979=AXIS2_PLACEMENT_3D ( 'NONE', #53949, #9432, #30941 ) ;
#15022=CYLINDRICAL_SURFACE ( 'NONE', #62479, 19.99999999999999645 ) ;
#15047=VERTEX_POINT ( 'NONE', #62209 ) ;
#15070=VERTEX_POINT ( 'NONE', #77710 ) ;
#15152=CARTESIAN_POINT ( 'NONE',  ( 38.04706783004212411, 44.99999999999999289, 7.000000000000000000 ) ) ;
#15175=ORIENTED_EDGE ( 'NONE', *, *, #81721, .T. ) ;
#15449=ADVANCED_FACE ( 'NONE', ( #18596, #72078, #88559 ), #94095, .F. ) ;
#15487=CARTESIAN_POINT ( 'NONE',  ( -0.07285406091746288171, 0.4131759111665360140, -9.500000000000000000 ) ) ;
#15488=EDGE_CURVE ( 'NONE', #66734, #11231, #20062, .T. ) ;
#15495=CIRCLE ( 'NONE', #28234, 0.4999999999999998890 ) ;
#15539=LINE ( 'NONE', #82530, #34600 ) ;
#15557=CIRCLE ( 'NONE', #71425, 2.500000000000002220 ) ;
#15617=AXIS2_PLACEMENT_3D ( 'NONE', #77617, #62116, #2156 ) ;
#15673=ORIENTED_EDGE ( 'NONE', *, *, #51915, .F. ) ;
#15702=ORIENTED_EDGE ( 'NONE', *, *, #79044, .T. ) ;
#15850=DIRECTION ( 'NONE',  ( 1.000000000000000000, 6.938893903907222067E-15, 0.000000000000000000 ) ) ;
#15877=CARTESIAN_POINT ( 'NONE',  ( 64.56412365047462742, 26.99999999999999645, 10.00000000000000000 ) ) ;
#15916=CARTESIAN_POINT ( 'NONE',  ( 66.56412365047464164, 26.99999999999998224, -9.500000000000000000 ) ) ;
#15928=ORIENTED_EDGE ( 'NONE', *, *, #348, .T. ) ;
#15953=LINE ( 'NONE', #1462, #81304 ) ;
#15993=CARTESIAN_POINT ( 'NONE',  ( 69.60148758828984228, -4.049828892140921146E-15, 9.500000000000000000 ) ) ;
#16001=CARTESIAN_POINT ( 'NONE',  ( 64.56412365047461321, -3.756725070333740926E-15, -7.000000000000000000 ) ) ;
#16030=VERTEX_POINT ( 'NONE', #61998 ) ;
#16099=DIRECTION ( 'NONE',  ( -0.000000000000000000, 1.000000000000000000, -0.000000000000000000 ) ) ;
#16101=DIRECTION ( 'NONE',  ( 1.000000000000000000, -5.818595309480553908E-17, 5.329070518200750605E-15 ) ) ;
#16107=DIRECTION ( 'NONE',  ( 1.000000000000000000, 0.000000000000000000, 0.000000000000000000 ) ) ;
#16208=DIRECTION ( 'NONE',  ( 0.000000000000000000, 0.000000000000000000, -1.000000000000000000 ) ) ;
#16221=EDGE_CURVE ( 'NONE', #40747, #83143, #53983, .T. ) ;
#16253=ORIENTED_EDGE ( 'NONE', *, *, #25653, .T. ) ;
#16297=EDGE_CURVE ( 'NONE', #10816, #68783, #50937, .T. ) ;
#16301=DIRECTION ( 'NONE',  ( -5.818595309480553908E-17, -1.000000000000000000, -0.000000000000000000 ) ) ;
#16319=SURFACE_STYLE_FILL_AREA ( #14857 ) ;
#16331=AXIS2_PLACEMENT_3D ( 'NONE', #985, #92448, #23972 ) ;
#16333=LINE ( 'NONE', #46816, #74445 ) ;
#16339=VECTOR ( 'NONE', #94279, 1000.000000000000000 ) ;
#16341=PLANE ( 'NONE',  #92788 ) ;
#16345=FACE_OUTER_BOUND ( 'NONE', #68791, .T. ) ;
#16346=CARTESIAN_POINT ( 'NONE',  ( 64.56412365047461321, 29.50000000000000000, -9.500000000000000000 ) ) ;
#16470=CIRCLE ( 'NONE', #29219, 0.5000000000000004441 ) ;
#16578=CARTESIAN_POINT ( 'NONE',  ( 17.35999999999999943, 37.99999999999997868, 9.500000000000000000 ) ) ;
#16719=ORIENTED_EDGE ( 'NONE', *, *, #71522, .F. ) ;
#16725=CARTESIAN_POINT ( 'NONE',  ( -27.43587634952538323, 44.49999999999997158, 10.00000000000000000 ) ) ;
#16744=ORIENTED_EDGE ( 'NONE', *, *, #65690, .T. ) ;
#16888=VECTOR ( 'NONE', #68464, 1000.000000000000000 ) ;
#17033=AXIS2_PLACEMENT_3D ( 'NONE', #27253, #4282, #65246 ) ;
#17097=DIRECTION ( 'NONE',  ( -1.000000000000000000, 0.000000000000000000, 0.000000000000000000 ) ) ;
#17194=VECTOR ( 'NONE', #4386, 1000.000000000000000 ) ;
#17206=CARTESIAN_POINT ( 'NONE',  ( -0.4427729075171641382, 14.61885305295417048, 9.500000000000000000 ) ) ;
#17284=DIRECTION ( 'NONE',  ( 1.000000000000000000, -5.818595309480553908E-17, 0.000000000000000000 ) ) ;
#17296=AXIS2_PLACEMENT_3D ( 'NONE', #43269, #73764, #36271 ) ;
#17330=DIRECTION ( 'NONE',  ( -0.000000000000000000, -0.000000000000000000, -1.000000000000000000 ) ) ;
#17331=AXIS2_PLACEMENT_3D ( 'NONE', #18602, #49567, #19578 ) ;
#17396=ORIENTED_EDGE ( 'NONE', *, *, #79500, .F. ) ;
#17420=CARTESIAN_POINT ( 'NONE',  ( 17.85999999999999233, 22.49999999999995026, 10.00000000000000000 ) ) ;
#17459=FACE_OUTER_BOUND ( 'NONE', #22656, .T. ) ;
#17553=LINE ( 'NONE', #1574, #49000 ) ;
#17574=ORIENTED_EDGE ( 'NONE', *, *, #36512, .T. ) ;
#17601=ORIENTED_EDGE ( 'NONE', *, *, #1722, .T. ) ;
#17616=AXIS2_PLACEMENT_3D ( 'NONE', #45127, #12663, #58655 ) ;
#17703=CARTESIAN_POINT ( 'NONE',  ( 2.618367889266248100E-15, 44.99999999999999289, -7.000000000000000000 ) ) ;
#17734=CARTESIAN_POINT ( 'NONE',  ( -27.43587634952537968, 11.50000000000000000, -9.500000000000000000 ) ) ;
#17759=ORIENTED_EDGE ( 'NONE', *, *, #45045, .F. ) ;
#17766=VECTOR ( 'NONE', #6273, 1000.000000000000000 ) ;
#17811=LINE ( 'NONE', #26280, #90681 ) ;
#17962=VECTOR ( 'NONE', #26921, 1000.000000000000000 ) ;
#17982=AXIS2_PLACEMENT_3D ( 'NONE', #83361, #61827, #84359 ) ;
#18019=CARTESIAN_POINT ( 'NONE',  ( 66.56412365047464164, 14.00000000000000888, 9.500000000000000000 ) ) ;
#18090=VERTEX_POINT ( 'NONE', #41743 ) ;
#18112=DIRECTION ( 'NONE',  ( -0.000000000000000000, 0.000000000000000000, -1.000000000000000000 ) ) ;
#18135=DIRECTION ( 'NONE',  ( 0.9848077530122084644, 0.1736481776669282495, 0.000000000000000000 ) ) ;
#18146=CARTESIAN_POINT ( 'NONE',  ( -27.43587634952537968, 29.50000000000000000, -10.00000000000000000 ) ) ;
#18198=LINE ( 'NONE', #48678, #2441 ) ;
#18199=DIRECTION ( 'NONE',  ( 0.000000000000000000, 0.000000000000000000, 1.000000000000000000 ) ) ;
#18217=ORIENTED_EDGE ( 'NONE', *, *, #81204, .F. ) ;
#18342=CARTESIAN_POINT ( 'NONE',  ( -0.4427729075171647488, 14.61885305295417758, -9.500000000000000000 ) ) ;
#18355=ORIENTED_EDGE ( 'NONE', *, *, #22774, .F. ) ;
#18401=AXIS2_PLACEMENT_3D ( 'NONE', #7257, #98777, #31212 ) ;
#18435=EDGE_CURVE ( 'NONE', #66580, #30184, #22484, .T. ) ;
#18477=CIRCLE ( 'NONE', #69577, 0.5000000000000004441 ) ;
#18488=VERTEX_POINT ( 'NONE', #34699 ) ;
#18505=CARTESIAN_POINT ( 'NONE',  ( 67.06412365047464164, 26.99999999999997868, -10.00000000000000000 ) ) ;
#18509=EDGE_CURVE ( 'NONE', #61145, #24437, #73559, .T. ) ;
#18596=FACE_BOUND ( 'NONE', #58065, .T. ) ;
#18602=CARTESIAN_POINT ( 'NONE',  ( 2.618367889266248100E-15, 44.99999999999999289, -7.000000000000000000 ) ) ;
#18618=AXIS2_PLACEMENT_3D ( 'NONE', #19740, #12728, #35223 ) ;
#18663=DIRECTION ( 'NONE',  ( -0.000000000000000000, -0.000000000000000000, -1.000000000000000000 ) ) ;
#18684=TOROIDAL_SURFACE ( 'NONE', #34643, 2.500000000000000888, 0.5000000000000000000 ) ;
#18767=DIRECTION ( 'NONE',  ( -1.000000000000000000, 0.000000000000000000, 0.000000000000000000 ) ) ;
#18773=FACE_OUTER_BOUND ( 'NONE', #31813, .T. ) ;
#18867=EDGE_CURVE ( 'NONE', #49892, #61653, #63841, .T. ) ;
#18908=EDGE_CURVE ( 'NONE', #60520, #82054, #97352, .T. ) ;
#18942=LINE ( 'NONE', #96926, #17962 ) ;
#18967=VERTEX_POINT ( 'NONE', #70150 ) ;
#18973=CARTESIAN_POINT ( 'NONE',  ( 12.26500600480480863, -7.132017415881208855E-16, 0.000000000000000000 ) ) ;
#19076=ADVANCED_FACE ( 'NONE', ( #78441 ), #94425, .T. ) ;
#19089=FACE_BOUND ( 'NONE', #47864, .T. ) ;
#19102=EDGE_LOOP ( 'NONE', ( #27958, #24021, #80086, #27171 ) ) ;
#19124=ORIENTED_EDGE ( 'NONE', *, *, #18908, .F. ) ;
#19145=ORIENTED_EDGE ( 'NONE', *, *, #73553, .F. ) ;
#19154=FACE_OUTER_BOUND ( 'NONE', #82665, .T. ) ;
#19189=ORIENTED_EDGE ( 'NONE', *, *, #94387, .T. ) ;
#19190=CYLINDRICAL_SURFACE ( 'NONE', #96214, 0.5000000000000000000 ) ;
#19192=ORIENTED_EDGE ( 'NONE', *, *, #20344, .F. ) ;
#19245=DIRECTION ( 'NONE',  ( -1.000000000000000000, 0.000000000000000000, 0.000000000000000000 ) ) ;
#19249=DIRECTION ( 'NONE',  ( 5.818595309480553908E-17, 1.000000000000000000, 0.000000000000000000 ) ) ;
#19262=ORIENTED_EDGE ( 'NONE', *, *, #69551, .F. ) ;
#19334=DIRECTION ( 'NONE',  ( -1.000000000000000000, 0.000000000000000000, 0.000000000000000000 ) ) ;
#19336=EDGE_LOOP ( 'NONE', ( #11417, #47132, #41714, #61142 ) ) ;
#19428=DIRECTION ( 'NONE',  ( -1.000000000000000000, 0.000000000000000000, 0.000000000000000000 ) ) ;
#19491=DIRECTION ( 'NONE',  ( 8.673617379884028570E-16, 1.000000000000000000, 0.000000000000000000 ) ) ;
#19499=EDGE_LOOP ( 'NONE', ( #86516, #85166, #5674, #34565 ) ) ;
#19519=CARTESIAN_POINT ( 'NONE',  ( 0.4195498155886330238, 0.5000000000000023315, 9.500000000000000000 ) ) ;
#19540=CARTESIAN_POINT ( 'NONE',  ( 17.35999999999999943, 37.99999999999997868, 10.00000000000000000 ) ) ;
#19578=DIRECTION ( 'NONE',  ( -1.000000000000000000, 0.000000000000000000, -0.000000000000000000 ) ) ;
#19582=ORIENTED_EDGE ( 'NONE', *, *, #24899, .T. ) ;
#19721=DIRECTION ( 'NONE',  ( -0.000000000000000000, -0.000000000000000000, -1.000000000000000000 ) ) ;
#19724=ORIENTED_EDGE ( 'NONE', *, *, #46856, .T. ) ;
#19740=CARTESIAN_POINT ( 'NONE',  ( 34.56412365047463453, 26.99999999999999645, 10.00000000000000000 ) ) ;
#19810=AXIS2_PLACEMENT_3D ( 'NONE', #43620, #28124, #58624 ) ;
#19891=CIRCLE ( 'NONE', #51877, 0.5000000000000004441 ) ;
#19939=ORIENTED_EDGE ( 'NONE', *, *, #63217, .T. ) ;
#20006=DIRECTION ( 'NONE',  ( -0.000000000000000000, -0.000000000000000000, -1.000000000000000000 ) ) ;
#20028=EDGE_CURVE ( 'NONE', #77584, #94846, #45115, .T. ) ;
#20062=LINE ( 'NONE', #34557, #55558 ) ;
#20098=EDGE_CURVE ( 'NONE', #56218, #63343, #53118, .T. ) ;
#20106=VERTEX_POINT ( 'NONE', #20785 ) ;
#20141=DIRECTION ( 'NONE',  ( -1.000000000000000000, 6.938893903907222067E-15, 0.000000000000000000 ) ) ;
#20171=AXIS2_PLACEMENT_3D ( 'NONE', #25424, #64367, #8918 ) ;
#20172=VERTEX_POINT ( 'NONE', #41824 ) ;
#20199=EDGE_CURVE ( 'NONE', #60520, #51757, #11794, .T. ) ;
#20200=DIRECTION ( 'NONE',  ( -0.000000000000000000, -0.000000000000000000, -1.000000000000000000 ) ) ;
#20237=LINE ( 'NONE', #51227, #4969 ) ;
#20319=ORIENTED_EDGE ( 'NONE', *, *, #67059, .T. ) ;
#20344=EDGE_CURVE ( 'NONE', #53120, #47516, #39955, .T. ) ;
#20371=LINE ( 'NONE', #81357, #72808 ) ;
#20467=EDGE_CURVE ( 'NONE', #1194, #35951, #49498, .T. ) ;
#20515=VERTEX_POINT ( 'NONE', #38137 ) ;
#20516=DIRECTION ( 'NONE',  ( -1.000000000000000000, 0.000000000000000000, 0.000000000000000000 ) ) ;
#20531=EDGE_LOOP ( 'NONE', ( #44330, #10130, #35029, #69999 ) ) ;
#20626=LINE ( 'NONE', #4650, #88788 ) ;
#20645=DIRECTION ( 'NONE',  ( -1.000000000000000000, 0.000000000000000000, 0.000000000000000000 ) ) ;
#20669=FACE_OUTER_BOUND ( 'NONE', #82579, .T. ) ;
#20723=CARTESIAN_POINT ( 'NONE',  ( 66.76470751278411342, 44.49999999999998579, -10.00000000000000000 ) ) ;
#20785=CARTESIAN_POINT ( 'NONE',  ( 38.04706783004212411, 44.99999999999998579, -7.000000000000000000 ) ) ;
#20789=CARTESIAN_POINT ( 'NONE',  ( 70.19910379943081580, 41.67447916666664298, 9.500000000000000000 ) ) ;
#20819=VERTEX_POINT ( 'NONE', #71584 ) ;
#20830=EDGE_LOOP ( 'NONE', ( #13331, #75595, #90781, #3664 ) ) ;
#20847=CIRCLE ( 'NONE', #46403, 20.00000000000000000 ) ;
#20900=ORIENTED_EDGE ( 'NONE', *, *, #58413, .F. ) ;
#20931=TOROIDAL_SURFACE ( 'NONE', #9724, 2.500000000000000888, 0.5000000000000000000 ) ;
#21012=CARTESIAN_POINT ( 'NONE',  ( -27.43587634952537968, 22.49999999999998934, -10.00000000000000000 ) ) ;
#21090=( LENGTH_UNIT ( ) NAMED_UNIT ( * ) SI_UNIT ( .MILLI., .METRE. ) );
#21123=ORIENTED_EDGE ( 'NONE', *, *, #57955, .F. ) ;
#21141=AXIS2_PLACEMENT_3D ( 'NONE', #24910, #48862, #1923 ) ;
#21147=UNCERTAINTY_MEASURE_WITH_UNIT (LENGTH_MEASURE( 1.000000000000000082E-05 ), #21090, 'distance_accuracy_value', 'NONE');
#21219=DIRECTION ( 'NONE',  ( 0.000000000000000000, -1.000000000000000000, 0.000000000000000000 ) ) ;
#21229=ADVANCED_FACE ( 'NONE', ( #38018 ), #76982, .F. ) ;
#21273=CARTESIAN_POINT ( 'NONE',  ( 17.35999999999999943, 37.99999999999997868, 10.00000000000000000 ) ) ;
#21287=AXIS2_PLACEMENT_3D ( 'NONE', #24434, #70418, #24925 ) ;
#21320=EDGE_LOOP ( 'NONE', ( #72284, #83297, #2052, #69275, #2765, #95909, #34381 ) ) ;
#21341=DIRECTION ( 'NONE',  ( -0.000000000000000000, -0.000000000000000000, -1.000000000000000000 ) ) ;
#21377=CARTESIAN_POINT ( 'NONE',  ( 2.618367889266248100E-15, 44.99999999999999289, -7.000000000000000000 ) ) ;
#21391=CIRCLE ( 'NONE', #80483, 3.500000000000003109 ) ;
#21481=LINE ( 'NONE', #36483, #16888 ) ;
#21522=EDGE_CURVE ( 'NONE', #20172, #18488, #97497, .T. ) ;
#21588=ORIENTED_EDGE ( 'NONE', *, *, #45490, .F. ) ;
#21592=VECTOR ( 'NONE', #32260, 1000.000000000000000 ) ;
#21621=VECTOR ( 'NONE', #35472, 1000.000000000000000 ) ;
#21639=LINE ( 'NONE', #6623, #73505 ) ;
#21736=PLANE ( 'NONE',  #45570 ) ;
#21752=CARTESIAN_POINT ( 'NONE',  ( 66.76470751278411342, 40.99999999999997868, 10.00000000000000000 ) ) ;
#21779=DIRECTION ( 'NONE',  ( -0.000000000000000000, -0.000000000000000000, -1.000000000000000000 ) ) ;
#21789=AXIS2_PLACEMENT_3D ( 'NONE', #4062, #58519, #87546 ) ;
#21815=ORIENTED_EDGE ( 'NONE', *, *, #80132, .F. ) ;
#21842=EDGE_LOOP ( 'NONE', ( #86581, #52208, #56156, #92476 ) ) ;
#21857=FILL_AREA_STYLE_COLOUR ( '', #51848 ) ;
#21867=FACE_OUTER_BOUND ( 'NONE', #73480, .T. ) ;
#21883=AXIS2_PLACEMENT_3D ( 'NONE', #53197, #76197, #91692 ) ;
#21924=ORIENTED_EDGE ( 'NONE', *, *, #3766, .F. ) ;
#21940=EDGE_CURVE ( 'NONE', #25854, #50813, #42844, .T. ) ;
#22027=DIRECTION ( 'NONE',  ( 1.000000000000000000, 0.000000000000000000, 0.000000000000000000 ) ) ;
#22089=( NAMED_UNIT ( * ) SI_UNIT ( $, .STERADIAN. ) SOLID_ANGLE_UNIT ( ) );
#22103=PLANE ( 'NONE',  #92731 ) ;
#22105=CARTESIAN_POINT ( 'NONE',  ( 66.56412365047464164, 26.99999999999998224, 10.00000000000000000 ) ) ;
#22113=VERTEX_POINT ( 'NONE', #27827 ) ;
#22130=DIRECTION ( 'NONE',  ( -1.000000000000000000, 5.818595309480552676E-17, -0.000000000000000000 ) ) ;
#22199=ADVANCED_FACE ( 'NONE', ( #71861 ), #95774, .T. ) ;
#22214=ORIENTED_EDGE ( 'NONE', *, *, #64320, .T. ) ;
#22215=FACE_OUTER_BOUND ( 'NONE', #46547, .T. ) ;
#22274=AXIS2_PLACEMENT_3D ( 'NONE', #6193, #20200, #36698 ) ;
#22297=CARTESIAN_POINT ( 'NONE',  ( 17.72850354356589619, 33.99078749795486942, 10.00000000000000000 ) ) ;
#22350=ORIENTED_EDGE ( 'NONE', *, *, #47634, .T. ) ;
#22412=AXIS2_PLACEMENT_3D ( 'NONE', #32074, #24114, #69118 ) ;
#22436=ORIENTED_EDGE ( 'NONE', *, *, #10761, .F. ) ;
#22484=CIRCLE ( 'NONE', #22274, 6.499999999999995559 ) ;
#22656=EDGE_LOOP ( 'NONE', ( #25323, #92039, #66649, #53288, #43791, #62256, #50079, #38554 ) ) ;
#22707=CYLINDRICAL_SURFACE ( 'NONE', #36597, 19.99999999999999645 ) ;
#22774=EDGE_CURVE ( 'NONE', #69260, #83143, #38795, .T. ) ;
#22804=ORIENTED_EDGE ( 'NONE', *, *, #4631, .T. ) ;
#22850=ADVANCED_FACE ( 'NONE', ( #81212 ), #64222, .F. ) ;
#22860=DIRECTION ( 'NONE',  ( -5.818595309480553908E-17, -1.000000000000000000, -0.000000000000000000 ) ) ;
#22911=EDGE_CURVE ( 'NONE', #35183, #45903, #4243, .T. ) ;
#23051=CIRCLE ( 'NONE', #45361, 0.5000000000000004441 ) ;
#23065=ADVANCED_FACE ( 'NONE', ( #41273 ), #24057, .T. ) ;
#23080=CARTESIAN_POINT ( 'NONE',  ( 64.56412365047462742, 26.99999999999999645, -10.00000000000000000 ) ) ;
#23097=DIRECTION ( 'NONE',  ( -1.000000000000000000, 5.782411586589362323E-17, -0.000000000000000000 ) ) ;
#23104=STYLED_ITEM ( 'NONE', ( #46803 ), #30996 ) ;
#23172=CARTESIAN_POINT ( 'NONE',  ( 34.56412365047463453, 13.99999999999999645, 9.500000000000000000 ) ) ;
#23198=DIRECTION ( 'NONE',  ( -0.000000000000000000, -0.000000000000000000, -1.000000000000000000 ) ) ;
#23222=PRODUCT_CONTEXT ( 'NONE', #26983, 'mechanical' ) ;
#23351=DIRECTION ( 'NONE',  ( -1.000000000000000000, 0.000000000000000000, 0.000000000000000000 ) ) ;
#23422=DIRECTION ( 'NONE',  ( 0.000000000000000000, -1.000000000000000000, 0.000000000000000000 ) ) ;
#23424=LINE ( 'NONE', #67430, #42857 ) ;
#23426=ORIENTED_EDGE ( 'NONE', *, *, #38954, .T. ) ;
#23439=ORIENTED_EDGE ( 'NONE', *, *, #16221, .T. ) ;
#23450=CIRCLE ( 'NONE', #61748, 19.99999999999999645 ) ;
#23457=DIRECTION ( 'NONE',  ( 0.000000000000000000, 1.000000000000000000, 0.000000000000000000 ) ) ;
#23501=DIRECTION ( 'NONE',  ( -5.818595309480553908E-17, -1.000000000000000000, -0.000000000000000000 ) ) ;
#23622=CARTESIAN_POINT ( 'NONE',  ( 12.26500600480480863, -7.132017415881208855E-16, 0.000000000000000000 ) ) ;
#23627=AXIS2_PLACEMENT_3D ( 'NONE', #49689, #3728, #34189 ) ;
#23641=DIRECTION ( 'NONE',  ( -5.818595309480553908E-17, -1.000000000000000000, -0.000000000000000000 ) ) ;
#23717=ADVANCED_FACE ( 'NONE', ( #36335 ), #57506, .T. ) ;
#23818=ADVANCED_FACE ( 'NONE', ( #75810 ), #59321, .F. ) ;
#23929=VERTEX_POINT ( 'NONE', #98843 ) ;
#23968=EDGE_CURVE ( 'NONE', #75199, #42131, #52323, .T. ) ;
#23972=DIRECTION ( 'NONE',  ( 0.000000000000000000, 0.000000000000000000, -1.000000000000000000 ) ) ;
#24021=ORIENTED_EDGE ( 'NONE', *, *, #42833, .T. ) ;
#24057=TOROIDAL_SURFACE ( 'NONE', #51163, 1.499999999999996669, 0.5000000000000000000 ) ;
#24114=DIRECTION ( 'NONE',  ( 0.000000000000000000, 0.000000000000000000, -1.000000000000000000 ) ) ;
#24146=ORIENTED_EDGE ( 'NONE', *, *, #45124, .F. ) ;
#24159=VECTOR ( 'NONE', #72034, 1000.000000000000000 ) ;
#24189=CARTESIAN_POINT ( 'NONE',  ( 32.06412365047463453, 26.99999999999997868, -10.00000000000000000 ) ) ;
#24233=LINE ( 'NONE', #16725, #32826 ) ;
#24257=FACE_OUTER_BOUND ( 'NONE', #97602, .T. ) ;
#24298=VECTOR ( 'NONE', #67054, 1000.000000000000000 ) ;
#24301=LINE ( 'NONE', #76301, #21592 ) ;
#24314=DIRECTION ( 'NONE',  ( -1.000000000000000000, 5.782411586589362323E-17, 0.000000000000000000 ) ) ;
#24322=CIRCLE ( 'NONE', #84973, 0.5000000000000000000 ) ;
#24328=AXIS2_PLACEMENT_3D ( 'NONE', #44587, #43599, #37104 ) ;
#24339=DIRECTION ( 'NONE',  ( -1.000000000000000000, 5.818595309480552676E-17, -0.000000000000000000 ) ) ;
#24434=CARTESIAN_POINT ( 'NONE',  ( 34.56412365047464874, 29.50000000000000000, 9.500000000000000000 ) ) ;
#24437=VERTEX_POINT ( 'NONE', #88718 ) ;
#24470=AXIS2_PLACEMENT_3D ( 'NONE', #2912, #92407, #33363 ) ;
#24501=DIRECTION ( 'NONE',  ( -0.000000000000000000, -0.000000000000000000, -1.000000000000000000 ) ) ;
#24508=DIRECTION ( 'NONE',  ( 0.000000000000000000, 0.000000000000000000, 1.000000000000000000 ) ) ;
#24550=EDGE_CURVE ( 'NONE', #47516, #53120, #10044, .T. ) ;
#24612=ORIENTED_EDGE ( 'NONE', *, *, #31257, .F. ) ;
#24650=DIRECTION ( 'NONE',  ( 0.000000000000000000, 0.000000000000000000, 1.000000000000000000 ) ) ;
#24653=EDGE_LOOP ( 'NONE', ( #15175, #14070, #63843 ) ) ;
#24677=ADVANCED_FACE ( 'NONE', ( #89705 ), #5730, .T. ) ;
#24699=CARTESIAN_POINT ( 'NONE',  ( 66.76470751278411342, 40.99999999999997868, -10.00000000000000000 ) ) ;
#24722=CARTESIAN_POINT ( 'NONE',  ( -0.2838433074297238012, 13.12729635533385597, 10.00000000000000000 ) ) ;
#24827=PLANE ( 'NONE',  #41712 ) ;
#24837=DIRECTION ( 'NONE',  ( 0.000000000000000000, 0.000000000000000000, -1.000000000000000000 ) ) ;
#24843=ORIENTED_EDGE ( 'NONE', *, *, #1855, .F. ) ;
#24878=ORIENTED_EDGE ( 'NONE', *, *, #50729, .F. ) ;
#24899=EDGE_CURVE ( 'NONE', #53155, #78868, #90195, .T. ) ;
#24910=CARTESIAN_POINT ( 'NONE',  ( 0.4195498155886414615, 0.4999999999999994449, 9.500000000000000000 ) ) ;
#24925=DIRECTION ( 'NONE',  ( 0.000000000000000000, 0.000000000000000000, -1.000000000000000000 ) ) ;
#25022=CARTESIAN_POINT ( 'NONE',  ( 12.26500600480481040, 44.99999999999999289, 0.000000000000000000 ) ) ;
#25040=EDGE_LOOP ( 'NONE', ( #55127, #97613, #47375, #3239 ) ) ;
#25048=AXIS2_PLACEMENT_3D ( 'NONE', #58974, #27976, #96502 ) ;
#25049=LINE ( 'NONE', #25537, #55138 ) ;
#25073=LINE ( 'NONE', #86057, #7500 ) ;
#25097=DIRECTION ( 'NONE',  ( -0.9848077530122086864, -0.1736481776669272503, 0.000000000000000000 ) ) ;
#25102=DIRECTION ( 'NONE',  ( 0.000000000000000000, 0.000000000000000000, 1.000000000000000000 ) ) ;
#25147=VERTEX_POINT ( 'NONE', #18505 ) ;
#25173=AXIS2_PLACEMENT_3D ( 'NONE', #82753, #68750, #98287 ) ;
#25179=DIRECTION ( 'NONE',  ( -0.1736481776669272503, 0.9848077530122086864, -0.000000000000000000 ) ) ;
#25189=CIRCLE ( 'NONE', #50721, 1.999999999999996669 ) ;
#25266=VERTEX_POINT ( 'NONE', #18019 ) ;
#25281=ORIENTED_EDGE ( 'NONE', *, *, #92910, .T. ) ;
#25306=ADVANCED_FACE ( 'NONE', ( #13461 ), #51647, .T. ) ;
#25323=ORIENTED_EDGE ( 'NONE', *, *, #90908, .T. ) ;
#25345=EDGE_LOOP ( 'NONE', ( #71533, #10313, #56784, #43730, #50170, #44253, #71386 ) ) ;
#25424=CARTESIAN_POINT ( 'NONE',  ( -27.43587634952537968, 22.49999999999998934, -9.500000000000000000 ) ) ;
#25436=CARTESIAN_POINT ( 'NONE',  ( -27.43587634952537968, 22.49999999999998934, 9.500000000000000000 ) ) ;
#25453=LINE ( 'NONE', #9443, #78526 ) ;
#25496=DIRECTION ( 'NONE',  ( -0.000000000000000000, -0.000000000000000000, -1.000000000000000000 ) ) ;
#25537=CARTESIAN_POINT ( 'NONE',  ( 4.999999999999999112, 16.50982297312470592, 10.00000000000000000 ) ) ;
#25560=AXIS2_PLACEMENT_3D ( 'NONE', #25022, #40511, #86007 ) ;
#25653=EDGE_CURVE ( 'NONE', #60197, #46560, #2148, .T. ) ;
#25675=DIRECTION ( 'NONE',  ( 0.000000000000000000, 0.000000000000000000, -1.000000000000000000 ) ) ;
#25704=ORIENTED_EDGE ( 'NONE', *, *, #37254, .T. ) ;
#25709=DIRECTION ( 'NONE',  ( -1.000000000000000000, 0.000000000000000000, 0.000000000000000000 ) ) ;
#25726=ORIENTED_EDGE ( 'NONE', *, *, #416, .T. ) ;
#25729=CARTESIAN_POINT ( 'NONE',  ( 64.56412365047462742, 26.99999999999999645, 9.500000000000000000 ) ) ;
#25760=ORIENTED_EDGE ( 'NONE', *, *, #42026, .T. ) ;
#25807=DIRECTION ( 'NONE',  ( -1.000000000000000000, 0.000000000000000000, 0.000000000000000000 ) ) ;
#25854=VERTEX_POINT ( 'NONE', #11131 ) ;
#25878=FACE_OUTER_BOUND ( 'NONE', #53735, .T. ) ;
#25901=ORIENTED_EDGE ( 'NONE', *, *, #624, .T. ) ;
#25920=CARTESIAN_POINT ( 'NONE',  ( -0.2838433074297238012, 13.12729635533385597, 10.00000000000000000 ) ) ;
#25938=CARTESIAN_POINT ( 'NONE',  ( 34.56412365047464874, 29.50000000000000000, -10.00000000000000000 ) ) ;
#25948=VERTEX_POINT ( 'NONE', #40658 ) ;
#25965=AXIS2_PLACEMENT_3D ( 'NONE', #9390, #2410, #62375 ) ;
#26224=CARTESIAN_POINT ( 'NONE',  ( 64.56412365047461321, 29.50000000000000000, -10.00000000000000000 ) ) ;
#26239=ADVANCED_FACE ( 'NONE', ( #96118 ), #36090, .F. ) ;
#26280=CARTESIAN_POINT ( 'NONE',  ( 64.56412365047461321, 28.99999999999999645, 10.00000000000000000 ) ) ;
#26354=DIRECTION ( 'NONE',  ( -0.000000000000000000, -0.000000000000000000, -1.000000000000000000 ) ) ;
#26456=DIRECTION ( 'NONE',  ( 5.818595309480553908E-17, 1.000000000000000000, -0.000000000000000000 ) ) ;
#26610=EDGE_LOOP ( 'NONE', ( #65461, #56717, #53352, #61 ) ) ;
#26646=CYLINDRICAL_SURFACE ( 'NONE', #19810, 0.5000000000000004441 ) ;
#26684=EDGE_LOOP ( 'NONE', ( #62951, #75029, #24612, #66339 ) ) ;
#26685=ORIENTED_EDGE ( 'NONE', *, *, #65751, .T. ) ;
#26699=DIRECTION ( 'NONE',  ( -5.818595309480553908E-17, -1.000000000000000000, -0.000000000000000000 ) ) ;
#26730=CIRCLE ( 'NONE', #76209, 0.5000000000000004441 ) ;
#26787=VERTEX_POINT ( 'NONE', #78372 ) ;
#26876=EDGE_CURVE ( 'NONE', #53155, #44802, #30776, .T. ) ;
#26890=FACE_OUTER_BOUND ( 'NONE', #50394, .T. ) ;
#26916=DIRECTION ( 'NONE',  ( 1.000000000000000000, 0.000000000000000000, 0.000000000000000000 ) ) ;
#26921=DIRECTION ( 'NONE',  ( 1.000000000000000000, -0.000000000000000000, -0.000000000000000000 ) ) ;
#26983=APPLICATION_CONTEXT ( 'automotive_design' ) ;
#27058=FACE_OUTER_BOUND ( 'NONE', #87006, .T. ) ;
#27069=FACE_OUTER_BOUND ( 'NONE', #21320, .T. ) ;
#27097=DIRECTION ( 'NONE',  ( -0.000000000000000000, -0.000000000000000000, -1.000000000000000000 ) ) ;
#27104=DIRECTION ( 'NONE',  ( -0.000000000000000000, -0.000000000000000000, -1.000000000000000000 ) ) ;
#27144=DIRECTION ( 'NONE',  ( 0.000000000000000000, 0.000000000000000000, -1.000000000000000000 ) ) ;
#27171=ORIENTED_EDGE ( 'NONE', *, *, #80594, .T. ) ;
#27180=DIRECTION ( 'NONE',  ( 0.000000000000000000, -1.000000000000000000, 0.000000000000000000 ) ) ;
#27206=ORIENTED_EDGE ( 'NONE', *, *, #61925, .F. ) ;
#27212=EDGE_CURVE ( 'NONE', #25948, #67069, #3952, .T. ) ;
#27213=CARTESIAN_POINT ( 'NONE',  ( 70.68973184038034674, 41.77083333333331439, 10.00000000000000000 ) ) ;
#27253=CARTESIAN_POINT ( 'NONE',  ( -2.614810775378867191, 35.00346125376525919, -7.000000000000000888 ) ) ;
#27282=CARTESIAN_POINT ( 'NONE',  ( 2.618367889266248100E-15, 44.99999999999999289, 7.000000000000000000 ) ) ;
#27340=VECTOR ( 'NONE', #58361, 1000.000000000000000 ) ;
#27370=CIRCLE ( 'NONE', #12957, 0.5000000000000004441 ) ;
#27377=CARTESIAN_POINT ( 'NONE',  ( 34.56412365047464874, 11.99999999999999645, -7.000000000000000888 ) ) ;
#27405=DIRECTION ( 'NONE',  ( 5.818595309480553908E-17, 1.000000000000000000, -0.000000000000000000 ) ) ;
#27602=DIRECTION ( 'NONE',  ( -1.000000000000000000, 0.000000000000000000, 0.000000000000000000 ) ) ;
#27639=FACE_OUTER_BOUND ( 'NONE', #98814, .T. ) ;
#27691=VERTEX_POINT ( 'NONE', #98426 ) ;
#27710=DIRECTION ( 'NONE',  ( 1.000000000000000000, 0.000000000000000000, 0.000000000000000000 ) ) ;
#27712=EDGE_CURVE ( 'NONE', #45908, #15070, #11192, .T. ) ;
#27827=CARTESIAN_POINT ( 'NONE',  ( 34.56412365047464874, 11.99999999999999645, 9.500000000000000000 ) ) ;
#27832=ORIENTED_EDGE ( 'NONE', *, *, #50458, .T. ) ;
#27877=FACE_OUTER_BOUND ( 'NONE', #24653, .T. ) ;
#27931=AXIS2_PLACEMENT_3D ( 'NONE', #67341, #59335, #50356 ) ;
#27939=ORIENTED_EDGE ( 'NONE', *, *, #1615, .F. ) ;
#27951=VECTOR ( 'NONE', #19491, 1000.000000000000000 ) ;
#27958=ORIENTED_EDGE ( 'NONE', *, *, #30452, .F. ) ;
#27965=EDGE_CURVE ( 'NONE', #56218, #62023, #59077, .T. ) ;
#27966=DIRECTION ( 'NONE',  ( 0.000000000000000000, 6.938893903907222067E-15, 1.000000000000000000 ) ) ;
#27976=DIRECTION ( 'NONE',  ( -0.1736481776669272503, 0.9848077530122086864, -0.000000000000000000 ) ) ;
#28092=ORIENTED_EDGE ( 'NONE', *, *, #56558, .T. ) ;
#28096=ORIENTED_EDGE ( 'NONE', *, *, #94646, .F. ) ;
#28100=LINE ( 'NONE', #75583, #83416 ) ;
#28102=CARTESIAN_POINT ( 'NONE',  ( 17.85999999999999943, 37.99999999999997868, -9.500000000000000000 ) ) ;
#28113=ADVANCED_FACE ( 'NONE', ( #78001 ), #70510, .F. ) ;
#28124=DIRECTION ( 'NONE',  ( -0.000000000000000000, -0.000000000000000000, -1.000000000000000000 ) ) ;
#28138=CIRCLE ( 'NONE', #84047, 0.5000000000000000000 ) ;
#28146=AXIS2_PLACEMENT_3D ( 'NONE', #3269, #78773, #19245 ) ;
#28150=ORIENTED_EDGE ( 'NONE', *, *, #60958, .F. ) ;
#28231=VECTOR ( 'NONE', #53129, 1000.000000000000000 ) ;
#28234=AXIS2_PLACEMENT_3D ( 'NONE', #19519, #64992, #80519 ) ;
#28316=ORIENTED_EDGE ( 'NONE', *, *, #47634, .F. ) ;
#28354=AXIS2_PLACEMENT_3D ( 'NONE', #49561, #18112, #95577 ) ;
#28574=EDGE_CURVE ( 'NONE', #11231, #44163, #68202, .T. ) ;
#28589=VERTEX_POINT ( 'NONE', #20723 ) ;
#28657=VERTEX_POINT ( 'NONE', #52200 ) ;
#28688=ADVANCED_FACE ( 'NONE', ( #6701 ), #84432, .T. ) ;
#28735=AXIS2_PLACEMENT_3D ( 'NONE', #84124, #1127, #31589 ) ;
#28818=DIRECTION ( 'NONE',  ( 0.9752498888222641549, -0.2211055276381879986, 0.000000000000000000 ) ) ;
#28828=EDGE_CURVE ( 'NONE', #68783, #3546, #79303, .T. ) ;
#28965=DIRECTION ( 'NONE',  ( 0.000000000000000000, 0.000000000000000000, -1.000000000000000000 ) ) ;
#28975=FACE_OUTER_BOUND ( 'NONE', #92677, .T. ) ;
#28994=CARTESIAN_POINT ( 'NONE',  ( 70.19910379943080159, 41.67447916666664298, -9.500000000000000000 ) ) ;
#29117=EDGE_CURVE ( 'NONE', #57472, #28657, #15539, .T. ) ;
#29141=EDGE_LOOP ( 'NONE', ( #19724, #82796, #75015, #15673 ) ) ;
#29218=EDGE_LOOP ( 'NONE', ( #71486, #33139, #38912, #70482 ) ) ;
#29219=AXIS2_PLACEMENT_3D ( 'NONE', #70338, #79789, #24837 ) ;
#29249=ADVANCED_FACE ( 'NONE', ( #51543 ), #96886, .T. ) ;
#29252=VERTEX_POINT ( 'NONE', #76998 ) ;
#29255=CYLINDRICAL_SURFACE ( 'NONE', #25173, 0.5000000000000004441 ) ;
#29311=DIRECTION ( 'NONE',  ( 0.2211055276381909129, 0.9752498888222635998, -0.000000000000000000 ) ) ;
#29341=FACE_OUTER_BOUND ( 'NONE', #39661, .T. ) ;
#29373=CARTESIAN_POINT ( 'NONE',  ( 26.00000000000000355, 35.99999999999997158, 7.000000000000000888 ) ) ;
#29675=AXIS2_PLACEMENT_3D ( 'NONE', #54190, #16208, #46691 ) ;
#29687=DIRECTION ( 'NONE',  ( -1.000000000000000000, 5.782411586589362323E-17, 0.000000000000000000 ) ) ;
#29695=CARTESIAN_POINT ( 'NONE',  ( 38.04706783004212411, 12.00000000000001066, -7.000000000000000000 ) ) ;
#29756=LINE ( 'NONE', #60264, #68435 ) ;
#29838=CARTESIAN_POINT ( 'NONE',  ( 38.04706783004212411, 44.99999999999999289, 7.000000000000000000 ) ) ;
#29846=FACE_OUTER_BOUND ( 'NONE', #66368, .T. ) ;
#29849=CIRCLE ( 'NONE', #98573, 0.5000000000000004441 ) ;
#29865=LINE ( 'NONE', #59378, #67135 ) ;
#29872=CIRCLE ( 'NONE', #98584, 1.500000000000001332 ) ;
#30049=ORIENTED_EDGE ( 'NONE', *, *, #97151, .T. ) ;
#30055=CARTESIAN_POINT ( 'NONE',  ( 17.35999999999999943, 33.99999999999997158, -9.500000000000000000 ) ) ;
#30071=CARTESIAN_POINT ( 'NONE',  ( 38.04706783004212411, 12.00000000000001066, 7.000000000000000000 ) ) ;
#30090=LINE ( 'NONE', #37126, #3904 ) ;
#30125=ORIENTED_EDGE ( 'NONE', *, *, #67305, .T. ) ;
#30143=DIRECTION ( 'NONE',  ( 0.000000000000000000, -1.000000000000000000, 0.000000000000000000 ) ) ;
#30184=VERTEX_POINT ( 'NONE', #10338 ) ;
#30209=FACE_OUTER_BOUND ( 'NONE', #56388, .T. ) ;
#30263=AXIS2_PLACEMENT_3D ( 'NONE', #82846, #68843, #23351 ) ;
#30314=ORIENTED_EDGE ( 'NONE', *, *, #11238, .T. ) ;
#30360=DIRECTION ( 'NONE',  ( 1.000000000000000000, -0.000000000000000000, 0.000000000000000000 ) ) ;
#30452=EDGE_CURVE ( 'NONE', #39764, #20515, #44319, .T. ) ;
#30519=DIRECTION ( 'NONE',  ( -0.000000000000000000, -0.000000000000000000, -1.000000000000000000 ) ) ;
#30548=CARTESIAN_POINT ( 'NONE',  ( 17.85999999999999588, 33.98752635800203592, 10.00000000000000000 ) ) ;
#30776=LINE ( 'NONE', #53789, #84513 ) ;
#30890=B_SPLINE_CURVE_WITH_KNOTS ( 'NONE', 3,
 ( #90773, #22297, #68778, #45276, #91264, #6789 ),
 .UNSPECIFIED., .F., .F.,
 ( 4, 2, 4 ),
 ( -2.009308255746759193E-05, 0.0003744380149044889881, 0.0007689691123664455646 ),
 .UNSPECIFIED. ) ;
#30921=CYLINDRICAL_SURFACE ( 'NONE', #48311, 0.5000000000000004441 ) ;
#30941=DIRECTION ( 'NONE',  ( 5.818595309480553908E-17, 1.000000000000000000, 0.000000000000000000 ) ) ;
#30996=ADVANCED_BREP_SHAPE_REPRESENTATION ( '', ( #41283, #27931 ), #96613 ) ;
#31016=CIRCLE ( 'NONE', #56503, 0.5000000000000000000 ) ;
#31033=ORIENTED_EDGE ( 'NONE', *, *, #18908, .T. ) ;
#31051=EDGE_CURVE ( 'NONE', #86750, #47321, #29872, .T. ) ;
#31168=ADVANCED_FACE ( 'NONE', ( #72880 ), #55436, .T. ) ;
#31193=LINE ( 'NONE', #69214, #84294 ) ;
#31196=DIRECTION ( 'NONE',  ( 0.000000000000000000, 0.000000000000000000, 1.000000000000000000 ) ) ;
#31202=DIRECTION ( 'NONE',  ( -0.000000000000000000, -0.000000000000000000, -1.000000000000000000 ) ) ;
#31212=DIRECTION ( 'NONE',  ( -1.000000000000000000, 0.000000000000000000, 0.000000000000000000 ) ) ;
#31257=EDGE_CURVE ( 'NONE', #18488, #11195, #13966, .T. ) ;
#31274=ORIENTED_EDGE ( 'NONE', *, *, #27212, .T. ) ;
#31300=SURFACE_SIDE_STYLE ('',( #16319 ) ) ;
#31395=ORIENTED_EDGE ( 'NONE', *, *, #97920, .F. ) ;
#31481=DIRECTION ( 'NONE',  ( -1.000000000000000000, 0.000000000000000000, 0.000000000000000000 ) ) ;
#31521=ORIENTED_EDGE ( 'NONE', *, *, #37520, .T. ) ;
#31562=ORIENTED_EDGE ( 'NONE', *, *, #34474, .T. ) ;
#31578=CARTESIAN_POINT ( 'NONE',  ( 66.76470751278411342, 40.99999999999997868, 9.500000000000000000 ) ) ;
#31589=DIRECTION ( 'NONE',  ( -1.000000000000000000, 0.000000000000000000, 0.000000000000000000 ) ) ;
#31652=EDGE_CURVE ( 'NONE', #50813, #68545, #14876, .T. ) ;
#31684=CARTESIAN_POINT ( 'NONE',  ( 0.4195498155886419056, 0.4999999999999970579, -9.500000000000000000 ) ) ;
#31694=FACE_OUTER_BOUND ( 'NONE', #59181, .T. ) ;
#31706=DIRECTION ( 'NONE',  ( -0.000000000000000000, -0.000000000000000000, -1.000000000000000000 ) ) ;
#31729=DIRECTION ( 'NONE',  ( 0.000000000000000000, 0.000000000000000000, 1.000000000000000000 ) ) ;
#31757=ADVANCED_FACE ( 'NONE', ( #91842 ), #77310, .T. ) ;
#31782=DIRECTION ( 'NONE',  ( 5.782411586589362323E-17, 1.000000000000000000, -0.000000000000000000 ) ) ;
#31795=DIRECTION ( 'NONE',  ( 0.9752498888222641549, -0.2211055276381879986, 3.469446951953568040E-15 ) ) ;
#31813=EDGE_LOOP ( 'NONE', ( #97633, #15702, #7040, #61080, #25704, #19582, #62640, #36724 ) ) ;
#31881=EDGE_CURVE ( 'NONE', #37315, #1778, #25189, .T. ) ;
#31963=EDGE_CURVE ( 'NONE', #41634, #25948, #17811, .T. ) ;
#31981=DIRECTION ( 'NONE',  ( 0.000000000000000000, 0.000000000000000000, -1.000000000000000000 ) ) ;
#32000=EDGE_CURVE ( 'NONE', #92229, #44802, #40320, .T. ) ;
#32009=ADVANCED_FACE ( 'NONE', ( #78301 ), #71311, .T. ) ;
#32074=CARTESIAN_POINT ( 'NONE',  ( 26.00000000000000355, 35.99999999999997158, -7.000000000000000000 ) ) ;
#32110=ORIENTED_EDGE ( 'NONE', *, *, #74171, .F. ) ;
#32260=DIRECTION ( 'NONE',  ( 0.000000000000000000, -1.000000000000000000, 0.000000000000000000 ) ) ;
#32267=FACE_OUTER_BOUND ( 'NONE', #80814, .T. ) ;
#32286=ORIENTED_EDGE ( 'NONE', *, *, #62760, .F. ) ;
#32294=DIRECTION ( 'NONE',  ( 0.000000000000000000, 0.000000000000000000, 1.000000000000000000 ) ) ;
#32298=DIRECTION ( 'NONE',  ( 5.782411586589362323E-17, 1.000000000000000000, -0.000000000000000000 ) ) ;
#32352=ORIENTED_EDGE ( 'NONE', *, *, #55136, .T. ) ;
#32424=DIRECTION ( 'NONE',  ( -1.000000000000000000, 0.000000000000000000, 0.000000000000000000 ) ) ;
#32498=ORIENTED_EDGE ( 'NONE', *, *, #46856, .F. ) ;
#32529=ORIENTED_EDGE ( 'NONE', *, *, #40896, .T. ) ;
#32531=CARTESIAN_POINT ( 'NONE',  ( 67.06412365047464164, 26.99999999999998224, 10.00000000000000000 ) ) ;
#32559=EDGE_CURVE ( 'NONE', #11334, #77048, #56146, .T. ) ;
#32670=DIRECTION ( 'NONE',  ( -0.1736481776669272503, 0.9848077530122086864, 0.000000000000000000 ) ) ;
#32709=EDGE_LOOP ( 'NONE', ( #19939, #97091 ) ) ;
#32771=FACE_OUTER_BOUND ( 'NONE', #19499, .T. ) ;
#32809=EDGE_LOOP ( 'NONE', ( #14441, #74905, #8513, #8533 ) ) ;
#32826=VECTOR ( 'NONE', #54700, 1000.000000000000000 ) ;
#32848=ORIENTED_EDGE ( 'NONE', *, *, #58296, .F. ) ;
#32919=CARTESIAN_POINT ( 'NONE',  ( 17.35999999999999943, 33.99999999999997158, -9.500000000000000000 ) ) ;
#32956=DIRECTION ( 'NONE',  ( -0.1736481776669272503, 0.9848077530122086864, 0.000000000000000000 ) ) ;
#32972=ADVANCED_FACE ( 'NONE', ( #68822 ), #354, .F. ) ;
#32976=FACE_OUTER_BOUND ( 'NONE', #64772, .T. ) ;
#33037=DIRECTION ( 'NONE',  ( -5.818595309480553908E-17, -1.000000000000000000, -0.000000000000000000 ) ) ;
#33055=DIRECTION ( 'NONE',  ( 0.000000000000000000, 0.000000000000000000, 1.000000000000000000 ) ) ;
#33064=CIRCLE ( 'NONE', #52203, 2.500000000000002220 ) ;
#33075=LINE ( 'NONE', #63571, #79735 ) ;
#33139=ORIENTED_EDGE ( 'NONE', *, *, #29117, .F. ) ;
#33363=DIRECTION ( 'NONE',  ( -1.000000000000000000, 0.000000000000000000, 0.000000000000000000 ) ) ;
#33383=ORIENTED_EDGE ( 'NONE', *, *, #94387, .F. ) ;
#33404=EDGE_CURVE ( 'NONE', #23929, #62689, #20237, .T. ) ;
#33434=ORIENTED_EDGE ( 'NONE', *, *, #18435, .T. ) ;
#33513=VECTOR ( 'NONE', #58817, 1000.000000000000000 ) ;
#33517=DIRECTION ( 'NONE',  ( -0.000000000000000000, -0.000000000000000000, -1.000000000000000000 ) ) ;
#33553=ORIENTED_EDGE ( 'NONE', *, *, #41019, .T. ) ;
#33587=VECTOR ( 'NONE', #19721, 1000.000000000000000 ) ;
#33594=DIRECTION ( 'NONE',  ( -1.000000000000000000, 0.000000000000000000, 0.000000000000000000 ) ) ;
#33596=ORIENTED_EDGE ( 'NONE', *, *, #33404, .F. ) ;
#33641=PLANE ( 'NONE',  #29675 ) ;
#33717=ORIENTED_EDGE ( 'NONE', *, *, #9261, .T. ) ;
#33740=CIRCLE ( 'NONE', #52892, 0.5000000000000004441 ) ;
#33809=ORIENTED_EDGE ( 'NONE', *, *, #44112, .F. ) ;
#33848=AXIS2_PLACEMENT_3D ( 'NONE', #76470, #38484, #77440 ) ;
#33853=DIRECTION ( 'NONE',  ( -1.000000000000000000, 3.556618985922298287E-15, 0.000000000000000000 ) ) ;
#33872=EDGE_CURVE ( 'NONE', #66451, #10816, #1105, .T. ) ;
#33889=CIRCLE ( 'NONE', #83452, 0.5000000000000066613 ) ;
#33921=DIRECTION ( 'NONE',  ( -1.000000000000000000, 0.000000000000000000, 0.000000000000000000 ) ) ;
#34042=CARTESIAN_POINT ( 'NONE',  ( 64.56412365047461321, 11.99999999999999467, -9.500000000000000000 ) ) ;
#34070=AXIS2_PLACEMENT_3D ( 'NONE', #77165, #14722, #223 ) ;
#34071=PLANE ( 'NONE',  #17331 ) ;
#34171=ADVANCED_FACE ( 'NONE', ( #89375 ), #20931, .T. ) ;
#34189=DIRECTION ( 'NONE',  ( 1.000000000000000000, 0.000000000000000000, 0.000000000000000000 ) ) ;
#34262=CARTESIAN_POINT ( 'NONE',  ( 2.241241388159942801E-47, 3.851859888774471706E-31, -7.000000000000000000 ) ) ;
#34290=ADVANCED_FACE ( 'NONE', ( #29846, #36378 ), #91845, .F. ) ;
#34307=ORIENTED_EDGE ( 'NONE', *, *, #51780, .F. ) ;
#34340=DIRECTION ( 'NONE',  ( 0.000000000000000000, 0.000000000000000000, -1.000000000000000000 ) ) ;
#34354=DIRECTION ( 'NONE',  ( 0.000000000000000000, 0.000000000000000000, 1.000000000000000000 ) ) ;
#34381=ORIENTED_EDGE ( 'NONE', *, *, #18509, .F. ) ;
#34418=AXIS2_PLACEMENT_3D ( 'NONE', #93453, #92462, #38989 ) ;
#34474=EDGE_CURVE ( 'NONE', #24437, #18090, #67366, .T. ) ;
#34494=EDGE_LOOP ( 'NONE', ( #92126, #95843, #96026, #22804 ) ) ;
#34555=ADVANCED_FACE ( 'NONE', ( #69339 ), #16341, .T. ) ;
#34557=CARTESIAN_POINT ( 'NONE',  ( 24.35999999999999233, 44.99999999999997158, 10.00000000000000000 ) ) ;
#34565=ORIENTED_EDGE ( 'NONE', *, *, #9261, .F. ) ;
#34588=CLOSED_SHELL ( 'NONE', ( #76087, #22850, #28688, #23065, #72063, #88141, #34290, #338, #62238, #73821, #77671, #75536, #15449, #85801, #31168, #70564, #36696, #79008, #26239, #32009, #93248, #8605, #40293, #39543, #45738, #48205, #53109, #62546, #40209, #21229, #34555, #91778, #77793, #54181, #23818, #70030, #93805, #3998, #28113, #34171, #8927, #97002, #29249, #7501, #4904, #37531, #85303, #64461, #25306, #1599, #14817, #78771, #5280, #38408, #75768, #6041, #84328, #40190, #5376, #19076, #24677, #34689, #67420, #2757, #1655, #22199, #87730, #46532, #23717, #49325, #35906, #61760, #55262, #32972, #92206, #31757, #73580, #71571, #47917, #94743, #92359 ) ) ;
#34600=VECTOR ( 'NONE', #67540, 1000.000000000000000 ) ;
#34638=DIRECTION ( 'NONE',  ( 6.938893903907221278E-15, 1.000000000000000000, 0.000000000000000000 ) ) ;
#34643=AXIS2_PLACEMENT_3D ( 'NONE', #93091, #9602, #46608 ) ;
#34651=DIRECTION ( 'NONE',  ( -0.000000000000000000, -0.000000000000000000, -1.000000000000000000 ) ) ;
#34653=EDGE_CURVE ( 'NONE', #295, #25266, #84805, .T. ) ;
#34689=ADVANCED_FACE ( 'NONE', ( #93308 ), #65657, .T. ) ;
#34693=VERTEX_POINT ( 'NONE', #48296 ) ;
#34699=CARTESIAN_POINT ( 'NONE',  ( 17.85999999999999588, 33.98752635800203592, -10.00000000000000000 ) ) ;
#34746=ORIENTED_EDGE ( 'NONE', *, *, #20028, .T. ) ;
#34773=CARTESIAN_POINT ( 'NONE',  ( 17.35999999999999943, 37.99999999999997868, 9.500000000000000000 ) ) ;
#34844=ORIENTED_EDGE ( 'NONE', *, *, #82507, .T. ) ;
#34875=LINE ( 'NONE', #51863, #80338 ) ;
#34881=CARTESIAN_POINT ( 'NONE',  ( 66.56412365047464164, 26.99999999999998224, -9.500000000000000000 ) ) ;
#34903=CARTESIAN_POINT ( 'NONE',  ( 12.26500600480481040, 44.99999999999999289, 0.000000000000000000 ) ) ;
#34923=AXIS2_PLACEMENT_3D ( 'NONE', #66395, #96929, #19428 ) ;
#34933=VECTOR ( 'NONE', #16301, 1000.000000000000000 ) ;
#34972=LINE ( 'NONE', #81956, #21621 ) ;
#35029=ORIENTED_EDGE ( 'NONE', *, *, #78782, .F. ) ;
#35052=CARTESIAN_POINT ( 'NONE',  ( -0.4957494408796453977, 15.11603861882761812, 10.00000000000000000 ) ) ;
#35060=VERTEX_POINT ( 'NONE', #42277 ) ;
#35102=FACE_OUTER_BOUND ( 'NONE', #68189, .T. ) ;
#35109=DIRECTION ( 'NONE',  ( 1.000000000000000000, 0.000000000000000000, 0.000000000000000000 ) ) ;
#35159=EDGE_CURVE ( 'NONE', #75802, #49611, #88883, .T. ) ;
#35183=VERTEX_POINT ( 'NONE', #58232 ) ;
#35206=CARTESIAN_POINT ( 'NONE',  ( -0.2838433074297238012, 13.12729635533385597, -9.500000000000000000 ) ) ;
#35218=CARTESIAN_POINT ( 'NONE',  ( 64.56412365047462742, 26.99999999999999645, 10.00000000000000000 ) ) ;
#35223=DIRECTION ( 'NONE',  ( -1.000000000000000000, 0.000000000000000000, 0.000000000000000000 ) ) ;
#35279=LINE ( 'NONE', #36275, #17766 ) ;
#35286=CIRCLE ( 'NONE', #38525, 19.99999999999999645 ) ;
#35316=ORIENTED_EDGE ( 'NONE', *, *, #69274, .T. ) ;
#35322=VERTEX_POINT ( 'NONE', #52238 ) ;
#35424=ORIENTED_EDGE ( 'NONE', *, *, #39326, .T. ) ;
#35472=DIRECTION ( 'NONE',  ( 0.000000000000000000, 0.000000000000000000, 1.000000000000000000 ) ) ;
#35515=VECTOR ( 'NONE', #89055, 1000.000000000000000 ) ;
#35543=AXIS2_PLACEMENT_3D ( 'NONE', #68943, #83938, #75447 ) ;
#35786=ORIENTED_EDGE ( 'NONE', *, *, #44034, .F. ) ;
#35874=DIRECTION ( 'NONE',  ( 0.000000000000000000, 1.000000000000000000, 0.000000000000000000 ) ) ;
#35906=ADVANCED_FACE ( 'NONE', ( #27058 ), #65543, .T. ) ;
#35949=AXIS2_PLACEMENT_3D ( 'NONE', #75738, #82746, #75244 ) ;
#35951=VERTEX_POINT ( 'NONE', #61009 ) ;
#35965=LINE ( 'NONE', #88976, #27951 ) ;
#35983=VERTEX_POINT ( 'NONE', #98561 ) ;
#36085=CARTESIAN_POINT ( 'NONE',  ( 67.06412365047464164, 26.99999999999997868, -9.500000000000000000 ) ) ;
#36090=CYLINDRICAL_SURFACE ( 'NONE', #54844, 19.99999999999999645 ) ;
#36127=CARTESIAN_POINT ( 'NONE',  ( 64.56412365047462742, 13.99999999999999467, 10.00000000000000000 ) ) ;
#36271=DIRECTION ( 'NONE',  ( 0.000000000000000000, -1.000000000000000000, 0.000000000000000000 ) ) ;
#36275=CARTESIAN_POINT ( 'NONE',  ( 38.04706783004212411, 44.99999999999999289, -7.000000000000000000 ) ) ;
#36335=FACE_OUTER_BOUND ( 'NONE', #59219, .T. ) ;
#36378=FACE_BOUND ( 'NONE', #683, .T. ) ;
#36425=DIRECTION ( 'NONE',  ( -1.000000000000000000, 0.000000000000000000, 0.000000000000000000 ) ) ;
#36482=PRODUCT_DEFINITION_CONTEXT ( 'detailed design', #98582, 'design' ) ;
#36483=CARTESIAN_POINT ( 'NONE',  ( 34.56412365047464874, 28.99999999999999645, 9.500000000000000000 ) ) ;
#36512=EDGE_CURVE ( 'NONE', #29252, #84180, #28138, .T. ) ;
#36521=ORIENTED_EDGE ( 'NONE', *, *, #59631, .F. ) ;
#36568=ORIENTED_EDGE ( 'NONE', *, *, #57583, .F. ) ;
#36597=AXIS2_PLACEMENT_3D ( 'NONE', #45194, #66714, #5727 ) ;
#36696=ADVANCED_FACE ( 'NONE', ( #82406 ), #60396, .T. ) ;
#36698=DIRECTION ( 'NONE',  ( -1.000000000000000000, 0.000000000000000000, 0.000000000000000000 ) ) ;
#36724=ORIENTED_EDGE ( 'NONE', *, *, #4446, .F. ) ;
#36749=CARTESIAN_POINT ( 'NONE',  ( 64.56412365047462742, 26.99999999999999645, 9.500000000000000000 ) ) ;
#36948=CIRCLE ( 'NONE', #6603, 0.5000000000000004441 ) ;
#37075=AXIS2_PLACEMENT_3D ( 'NONE', #20789, #88290, #88782 ) ;
#37104=DIRECTION ( 'NONE',  ( -1.000000000000000000, 0.000000000000000000, 0.000000000000000000 ) ) ;
#37126=CARTESIAN_POINT ( 'NONE',  ( 17.35999999999999943, 37.99999999999997868, 10.00000000000000000 ) ) ;
#37138=CARTESIAN_POINT ( 'NONE',  ( 0.000000000000000000, 0.000000000000000000, 9.500000000000000000 ) ) ;
#37164=FACE_BOUND ( 'NONE', #49477, .T. ) ;
#37226=DIRECTION ( 'NONE',  ( 0.000000000000000000, 0.000000000000000000, -1.000000000000000000 ) ) ;
#37250=DIRECTION ( 'NONE',  ( -1.000000000000000000, 0.000000000000000000, 0.000000000000000000 ) ) ;
#37254=EDGE_CURVE ( 'NONE', #295, #53155, #20371, .T. ) ;
#37315=VERTEX_POINT ( 'NONE', #41176 ) ;
#37416=CARTESIAN_POINT ( 'NONE',  ( 34.56412365047463453, 26.99999999999999645, 9.500000000000000000 ) ) ;
#37436=DIRECTION ( 'NONE',  ( 0.000000000000000000, 0.000000000000000000, 1.000000000000000000 ) ) ;
#37468=FACE_OUTER_BOUND ( 'NONE', #25040, .T. ) ;
#37520=EDGE_CURVE ( 'NONE', #20819, #67069, #4150, .T. ) ;
#37531=ADVANCED_FACE ( 'NONE', ( #39322 ), #71170, .T. ) ;
#37597=FACE_OUTER_BOUND ( 'NONE', #65605, .T. ) ;
#37677=ORIENTED_EDGE ( 'NONE', *, *, #54989, .F. ) ;
#37780=EDGE_LOOP ( 'NONE', ( #88439, #46502, #86736, #94231 ) ) ;
#37932=DIRECTION ( 'NONE',  ( 1.000000000000000000, -5.818595309480552676E-17, 0.000000000000000000 ) ) ;
#38018=FACE_OUTER_BOUND ( 'NONE', #97895, .T. ) ;
#38109=ORIENTED_EDGE ( 'NONE', *, *, #8903, .T. ) ;
#38127=EDGE_CURVE ( 'NONE', #51757, #78249, #15495, .T. ) ;
#38137=CARTESIAN_POINT ( 'NONE',  ( 70.19910379943081580, 41.67447916666664298, 10.00000000000000000 ) ) ;
#38179=CIRCLE ( 'NONE', #39742, 2.000000000000001776 ) ;
#38233=LINE ( 'NONE', #44228, #4131 ) ;
#38258=LINE ( 'NONE', #21273, #79391 ) ;
#38299=EDGE_CURVE ( 'NONE', #24437, #44141, #25073, .T. ) ;
#38321=AXIS2_PLACEMENT_3D ( 'NONE', #94111, #24650, #33594 ) ;
#38354=CARTESIAN_POINT ( 'NONE',  ( 67.06412365047464164, 14.00000000000001243, 9.500000000000000000 ) ) ;
#38408=ADVANCED_FACE ( 'NONE', ( #28975 ), #61776, .T. ) ;
#38484=DIRECTION ( 'NONE',  ( 0.000000000000000000, -1.000000000000000000, 0.000000000000000000 ) ) ;
#38525=AXIS2_PLACEMENT_3D ( 'NONE', #44811, #45316, #98847 ) ;
#38554=ORIENTED_EDGE ( 'NONE', *, *, #41817, .T. ) ;
#38557=VERTEX_POINT ( 'NONE', #15487 ) ;
#38568=ORIENTED_EDGE ( 'NONE', *, *, #55136, .F. ) ;
#38607=FACE_OUTER_BOUND ( 'NONE', #168, .T. ) ;
#38622=LINE ( 'NONE', #92110, #66957 ) ;
#38795=LINE ( 'NONE', #9274, #62280 ) ;
#38801=DIRECTION ( 'NONE',  ( 5.818595309480553908E-17, 1.000000000000000000, -0.000000000000000000 ) ) ;
#38805=CARTESIAN_POINT ( 'NONE',  ( 32.26500600480481040, 44.99999999999999289, 0.000000000000000000 ) ) ;
#38827=( NAMED_UNIT ( * ) PLANE_ANGLE_UNIT ( ) SI_UNIT ( $, .RADIAN. ) );
#38837=CARTESIAN_POINT ( 'NONE',  ( 17.35999999999999943, 37.99999999999997868, -7.000000000000000888 ) ) ;
#38843=AXIS2_PLACEMENT_3D ( 'NONE', #51134, #34638, #20141 ) ;
#38844=CARTESIAN_POINT ( 'NONE',  ( -0.2838433074297238012, 13.12729635533385597, -9.500000000000000000 ) ) ;
#38885=DIRECTION ( 'NONE',  ( -0.1059530667249615893, 0.9943711317468825195, 0.000000000000000000 ) ) ;
#38897=AXIS2_PLACEMENT_3D ( 'NONE', #81710, #81229, #19249 ) ;
#38912=ORIENTED_EDGE ( 'NONE', *, *, #94646, .T. ) ;
#38954=EDGE_CURVE ( 'NONE', #92057, #60197, #66865, .T. ) ;
#38957=ORIENTED_EDGE ( 'NONE', *, *, #20199, .F. ) ;
#38989=DIRECTION ( 'NONE',  ( 0.9848077530122084644, 0.1736481776669282495, 0.000000000000000000 ) ) ;
#39017=EDGE_LOOP ( 'NONE', ( #92758, #9366, #26685, #55729 ) ) ;
#39188=CARTESIAN_POINT ( 'NONE',  ( 64.56412365047461321, 11.49999999999999467, 10.00000000000000000 ) ) ;
#39198=AXIS2_PLACEMENT_3D ( 'NONE', #69328, #90832, #83834 ) ;
#39322=FACE_OUTER_BOUND ( 'NONE', #51887, .T. ) ;
#39326=EDGE_CURVE ( 'NONE', #63343, #25266, #33740, .T. ) ;
#39441=CIRCLE ( 'NONE', #21883, 2.500000000000002220 ) ;
#39528=AXIS2_PLACEMENT_3D ( 'NONE', #36085, #50102, #85779 ) ;
#39543=ADVANCED_FACE ( 'NONE', ( #85814 ), #24827, .T. ) ;
#39557=ORIENTED_EDGE ( 'NONE', *, *, #13597, .F. ) ;
#39604=FACE_OUTER_BOUND ( 'NONE', #26610, .T. ) ;
#39660=EDGE_CURVE ( 'NONE', #77584, #20106, #44965, .T. ) ;
#39661=EDGE_LOOP ( 'NONE', ( #74566, #73146, #9991, #14686 ) ) ;
#39726=CARTESIAN_POINT ( 'NONE',  ( -0.2838433074297238012, 13.12729635533385597, -10.00000000000000000 ) ) ;
#39742=AXIS2_PLACEMENT_3D ( 'NONE', #23172, #83163, #83660 ) ;
#39759=DIRECTION ( 'NONE',  ( 8.673617379884027583E-16, 1.000000000000000000, -0.000000000000000000 ) ) ;
#39764=VERTEX_POINT ( 'NONE', #89737 ) ;
#39878=EDGE_CURVE ( 'NONE', #67069, #61160, #76711, .T. ) ;
#39955=CIRCLE ( 'NONE', #22412, 1.500000000000001332 ) ;
#40006=CYLINDRICAL_SURFACE ( 'NONE', #58780, 4.000000000000003553 ) ;
#40163=CARTESIAN_POINT ( 'NONE',  ( -1.761054936948036165, 12.86682408883346440, -10.00000000000000000 ) ) ;
#40184=DIRECTION ( 'NONE',  ( -1.000000000000000000, 0.000000000000000000, 0.000000000000000000 ) ) ;
#40190=ADVANCED_FACE ( 'NONE', ( #49164 ), #5307, .T. ) ;
#40202=EDGE_LOOP ( 'NONE', ( #14821, #79860, #78718, #59081 ) ) ;
#40209=ADVANCED_FACE ( 'NONE', ( #31694 ), #48172, .F. ) ;
#40230=CYLINDRICAL_SURFACE ( 'NONE', #11806, 0.5000000000000004441 ) ;
#40250=CARTESIAN_POINT ( 'NONE',  ( -27.43587634952537968, 0.5000000000000038858, 10.00000000000000000 ) ) ;
#40254=ORIENTED_EDGE ( 'NONE', *, *, #60958, .T. ) ;
#40278=LINE ( 'NONE', #38805, #34933 ) ;
#40292=CARTESIAN_POINT ( 'NONE',  ( 34.56412365047463453, 26.99999999999999645, -9.500000000000000000 ) ) ;
#40293=ADVANCED_FACE ( 'NONE', ( #27639 ), #96156, .F. ) ;
#40302=AXIS2_PLACEMENT_3D ( 'NONE', #8308, #67831, #7332 ) ;
#40306=CARTESIAN_POINT ( 'NONE',  ( 69.60148758828985649, 0.4999999999999935052, 9.500000000000000000 ) ) ;
#40320=LINE ( 'NONE', #64757, #44209 ) ;
#40328=LINE ( 'NONE', #34262, #77061 ) ;
#40337=ORIENTED_EDGE ( 'NONE', *, *, #56390, .T. ) ;
#40399=CYLINDRICAL_SURFACE ( 'NONE', #25965, 1.500000000000001332 ) ;
#40511=DIRECTION ( 'NONE',  ( -5.818595309480553908E-17, -1.000000000000000000, -0.000000000000000000 ) ) ;
#40534=EDGE_CURVE ( 'NONE', #10816, #87399, #93139, .T. ) ;
#40542=ORIENTED_EDGE ( 'NONE', *, *, #65751, .F. ) ;
#40585=DIRECTION ( 'NONE',  ( 0.000000000000000000, 0.000000000000000000, 1.000000000000000000 ) ) ;
#40628=ORIENTED_EDGE ( 'NONE', *, *, #40896, .F. ) ;
#40658=CARTESIAN_POINT ( 'NONE',  ( 64.56412365047461321, 29.00000000000000355, 7.000000000000000000 ) ) ;
#40660=LINE ( 'NONE', #56157, #93884 ) ;
#40676=CARTESIAN_POINT ( 'NONE',  ( 17.85999999999999588, 37.99999999999997868, 10.00000000000000000 ) ) ;
#40689=DIRECTION ( 'NONE',  ( 0.000000000000000000, 0.000000000000000000, -1.000000000000000000 ) ) ;
#40747=VERTEX_POINT ( 'NONE', #54452 ) ;
#40777=( GEOMETRIC_REPRESENTATION_CONTEXT ( 3 ) GLOBAL_UNCERTAINTY_ASSIGNED_CONTEXT ( ( #21147 ) ) GLOBAL_UNIT_ASSIGNED_CONTEXT ( ( #21090, #51589, #22089 ) ) REPRESENTATION_CONTEXT ( 'NONE', 'WORKASPACE' ) );
#40814=DIRECTION ( 'NONE',  ( -0.000000000000000000, -0.000000000000000000, -1.000000000000000000 ) ) ;
#40860=ORIENTED_EDGE ( 'NONE', *, *, #16221, .F. ) ;
#40893=VERTEX_POINT ( 'NONE', #25938 ) ;
#40896=EDGE_CURVE ( 'NONE', #6556, #4006, #87901, .T. ) ;
#40974=ORIENTED_EDGE ( 'NONE', *, *, #32559, .F. ) ;
#41019=EDGE_CURVE ( 'NONE', #12064, #40893, #86637, .T. ) ;
#41152=ORIENTED_EDGE ( 'NONE', *, *, #69551, .T. ) ;
#41176=CARTESIAN_POINT ( 'NONE',  ( -2.283843307429720415, 13.12729635533385597, -9.500000000000000000 ) ) ;
#41181=FACE_OUTER_BOUND ( 'NONE', #19102, .T. ) ;
#41273=FACE_OUTER_BOUND ( 'NONE', #11336, .T. ) ;
#41283=MANIFOLD_SOLID_BREP ( 'Fillet3', #34588 ) ;
#41319=DIRECTION ( 'NONE',  ( -0.000000000000000000, -0.000000000000000000, -1.000000000000000000 ) ) ;
#41344=AXIS2_PLACEMENT_3D ( 'NONE', #52688, #66203, #83192 ) ;
#41561=ORIENTED_EDGE ( 'NONE', *, *, #91196, .T. ) ;
#41634=VERTEX_POINT ( 'NONE', #43474 ) ;
#41636=ORIENTED_EDGE ( 'NONE', *, *, #88613, .F. ) ;
#41641=PRESENTATION_STYLE_ASSIGNMENT (( #87112 ) ) ;
#41644=AXIS2_PLACEMENT_3D ( 'NONE', #79640, #5124, #43110 ) ;
#41658=DIRECTION ( 'NONE',  ( 0.000000000000000000, 0.000000000000000000, 1.000000000000000000 ) ) ;
#41712=AXIS2_PLACEMENT_3D ( 'NONE', #94778, #86305, #71310 ) ;
#41714=ORIENTED_EDGE ( 'NONE', *, *, #49558, .T. ) ;
#41743=CARTESIAN_POINT ( 'NONE',  ( 31.00000000000000355, 44.99999999999999289, -7.000000000000000000 ) ) ;
#41744=CIRCLE ( 'NONE', #97632, 1.500000000000001332 ) ;
#41753=CARTESIAN_POINT ( 'NONE',  ( 24.35999999999999233, 44.99999999999997868, -9.500000000000000000 ) ) ;
#41760=DIRECTION ( 'NONE',  ( -0.000000000000000000, -0.000000000000000000, -1.000000000000000000 ) ) ;
#41817=EDGE_CURVE ( 'NONE', #41634, #45908, #21481, .T. ) ;
#41824=CARTESIAN_POINT ( 'NONE',  ( -0.4427729075171647488, 14.61885305295417758, -10.00000000000000000 ) ) ;
#41848=ORIENTED_EDGE ( 'NONE', *, *, #49678, .F. ) ;
#41852=CARTESIAN_POINT ( 'NONE',  ( -2.614810775378867191, 35.00346125376525919, 10.00000000000000000 ) ) ;
#41881=DIRECTION ( 'NONE',  ( 1.000000000000000000, -0.000000000000000000, 0.000000000000000000 ) ) ;
#41909=EDGE_CURVE ( 'NONE', #86750, #85266, #98492, .T. ) ;
#41918=DIRECTION ( 'NONE',  ( 0.000000000000000000, 0.000000000000000000, -1.000000000000000000 ) ) ;
#42026=EDGE_CURVE ( 'NONE', #35183, #6556, #53627, .T. ) ;
#42127=CARTESIAN_POINT ( 'NONE',  ( -2.614810775378867191, 35.00346125376525919, 9.500000000000000000 ) ) ;
#42131=VERTEX_POINT ( 'NONE', #54423 ) ;
#42260=CARTESIAN_POINT ( 'NONE',  ( -27.43587634952537968, 22.49999999999998934, -10.00000000000000000 ) ) ;
#42277=CARTESIAN_POINT ( 'NONE',  ( -0.4957494408796453977, 15.11603861882761812, -9.500000000000000000 ) ) ;
#42352=CARTESIAN_POINT ( 'NONE',  ( 27.50000000000000355, 35.99999999999997158, 7.000000000000000888 ) ) ;
#42452=DIRECTION ( 'NONE',  ( -1.084202172485504434E-16, -1.000000000000000000, 0.000000000000000000 ) ) ;
#42606=SURFACE_SIDE_STYLE ('',( #11609 ) ) ;
#42608=FACE_OUTER_BOUND ( 'NONE', #93739, .T. ) ;
#42631=DIRECTION ( 'NONE',  ( 1.000000000000000000, 0.000000000000000000, 0.000000000000000000 ) ) ;
#42710=DIRECTION ( 'NONE',  ( -1.000000000000000000, 0.000000000000000000, 0.000000000000000000 ) ) ;
#42833=EDGE_CURVE ( 'NONE', #39764, #6556, #93591, .T. ) ;
#42844=LINE ( 'NONE', #95852, #33513 ) ;
#42857=VECTOR ( 'NONE', #37932, 1000.000000000000000 ) ;
#42870=ORIENTED_EDGE ( 'NONE', *, *, #30452, .T. ) ;
#42883=DIRECTION ( 'NONE',  ( -1.000000000000000000, 5.782411586589362323E-17, 0.000000000000000000 ) ) ;
#42904=VERTEX_POINT ( 'NONE', #71778 ) ;
#42917=LINE ( 'NONE', #4442, #78689 ) ;
#42927=EDGE_LOOP ( 'NONE', ( #88602, #64020, #82769, #19124 ) ) ;
#42970=ORIENTED_EDGE ( 'NONE', *, *, #50461, .T. ) ;
#43042=FACE_OUTER_BOUND ( 'NONE', #68737, .T. ) ;
#43057=DIRECTION ( 'NONE',  ( 1.000000000000000000, 0.000000000000000000, -0.000000000000000000 ) ) ;
#43110=DIRECTION ( 'NONE',  ( 0.000000000000000000, -1.000000000000000000, 0.000000000000000000 ) ) ;
#43119=CARTESIAN_POINT ( 'NONE',  ( 26.00000000000000355, 35.99999999999997158, 10.00000000000000000 ) ) ;
#43128=FACE_OUTER_BOUND ( 'NONE', #39017, .T. ) ;
#43165=ORIENTED_EDGE ( 'NONE', *, *, #40534, .F. ) ;
#43166=DIRECTION ( 'NONE',  ( 5.818595309480552676E-17, 1.000000000000000000, -0.000000000000000000 ) ) ;
#43228=DIRECTION ( 'NONE',  ( -0.000000000000000000, 0.000000000000000000, -1.000000000000000000 ) ) ;
#43257=CIRCLE ( 'NONE', #68833, 6.999999999999995559 ) ;
#43269=CARTESIAN_POINT ( 'NONE',  ( 34.56412365047464874, 11.49999999999999645, 9.500000000000000000 ) ) ;
#43316=ORIENTED_EDGE ( 'NONE', *, *, #81721, .F. ) ;
#43318=ORIENTED_EDGE ( 'NONE', *, *, #24899, .F. ) ;
#43446=EDGE_CURVE ( 'NONE', #25266, #60197, #53206, .T. ) ;
#43454=ORIENTED_EDGE ( 'NONE', *, *, #1268, .F. ) ;
#43460=CARTESIAN_POINT ( 'NONE',  ( 0.4195498155886412950, 0.5000000000000000000, -10.00000000000000000 ) ) ;
#43466=AXIS2_PLACEMENT_3D ( 'NONE', #63373, #41881, #34340 ) ;
#43474=CARTESIAN_POINT ( 'NONE',  ( 64.56412365047461321, 28.99999999999999645, 9.500000000000000000 ) ) ;
#43556=ORIENTED_EDGE ( 'NONE', *, *, #59631, .T. ) ;
#43599=DIRECTION ( 'NONE',  ( -0.000000000000000000, -0.000000000000000000, -1.000000000000000000 ) ) ;
#43620=CARTESIAN_POINT ( 'NONE',  ( 69.60148758828984228, 0.4999999999999982792, 10.00000000000000000 ) ) ;
#43637=CARTESIAN_POINT ( 'NONE',  ( 64.56412365047461321, 11.99999999999999467, 10.00000000000000000 ) ) ;
#43659=ORIENTED_EDGE ( 'NONE', *, *, #14598, .T. ) ;
#43704=DIRECTION ( 'NONE',  ( 1.000000000000000000, -5.818595309480553908E-17, 0.000000000000000000 ) ) ;
#43730=ORIENTED_EDGE ( 'NONE', *, *, #31652, .F. ) ;
#43791=ORIENTED_EDGE ( 'NONE', *, *, #4245, .F. ) ;
#43801=ORIENTED_EDGE ( 'NONE', *, *, #21522, .T. ) ;
#43903=ORIENTED_EDGE ( 'NONE', *, *, #14061, .T. ) ;
#44000=DIRECTION ( 'NONE',  ( -0.1927083333333330095, 0.9812560818990572198, -5.348730717595142060E-15 ) ) ;
#44007=AXIS2_PLACEMENT_3D ( 'NONE', #65128, #3673, #64627 ) ;
#44019=CARTESIAN_POINT ( 'NONE',  ( 34.56412365047463453, 26.99999999999999645, -10.00000000000000000 ) ) ;
#44034=EDGE_CURVE ( 'NONE', #85266, #66421, #79226, .T. ) ;
#44112=EDGE_CURVE ( 'NONE', #82054, #1778, #20626, .T. ) ;
#44135=CARTESIAN_POINT ( 'NONE',  ( 69.60148758828984228, 0.4999999999999960032, -10.00000000000000000 ) ) ;
#44141=VERTEX_POINT ( 'NONE', #3661 ) ;
#44146=EDGE_CURVE ( 'NONE', #22113, #83062, #51115, .T. ) ;
#44163=VERTEX_POINT ( 'NONE', #64129 ) ;
#44209=VECTOR ( 'NONE', #47801, 1000.000000000000000 ) ;
#44228=CARTESIAN_POINT ( 'NONE',  ( 17.35999999999999943, 33.99999999999997158, 10.00000000000000000 ) ) ;
#44253=ORIENTED_EDGE ( 'NONE', *, *, #74171, .T. ) ;
#44282=CARTESIAN_POINT ( 'NONE',  ( 32.56412365047463453, 26.99999999999998224, -9.500000000000000000 ) ) ;
#44319=CIRCLE ( 'NONE', #6013, 99.50000000000000000 ) ;
#44330=ORIENTED_EDGE ( 'NONE', *, *, #31257, .T. ) ;
#44353=EDGE_LOOP ( 'NONE', ( #33553, #33717, #47966, #622, #7301, #85995, #13451, #30314 ) ) ;
#44375=EDGE_LOOP ( 'NONE', ( #14454, #89639, #49472, #27206 ) ) ;
#44442=VERTEX_POINT ( 'NONE', #16578 ) ;
#44587=CARTESIAN_POINT ( 'NONE',  ( 34.56412365047463453, 26.99999999999999645, 10.00000000000000000 ) ) ;
#44612=AXIS2_PLACEMENT_3D ( 'NONE', #97501, #28965, #59468 ) ;
#44621=AXIS2_PLACEMENT_3D ( 'NONE', #2601, #3082, #33055 ) ;
#44628=EDGE_CURVE ( 'NONE', #35322, #93263, #69576, .T. ) ;
#44699=CARTESIAN_POINT ( 'NONE',  ( 34.56412365047464874, 11.99999999999999645, 7.000000000000000000 ) ) ;
#44700=ORIENTED_EDGE ( 'NONE', *, *, #20467, .F. ) ;
#44738=ORIENTED_EDGE ( 'NONE', *, *, #38127, .T. ) ;
#44802=VERTEX_POINT ( 'NONE', #9458 ) ;
#44811=CARTESIAN_POINT ( 'NONE',  ( -2.614810775378867191, 35.00346125376525919, 9.500000000000000000 ) ) ;
#44821=( NAMED_UNIT ( * ) SI_UNIT ( $, .STERADIAN. ) SOLID_ANGLE_UNIT ( ) );
#44852=CYLINDRICAL_SURFACE ( 'NONE', #91409, 0.5000000000000004441 ) ;
#44965=CIRCLE ( 'NONE', #3456, 19.99999999999999645 ) ;
#45045=EDGE_CURVE ( 'NONE', #75802, #69260, #76479, .T. ) ;
#45071=AXIS2_PLACEMENT_3D ( 'NONE', #2687, #79141, #10652 ) ;
#45115=LINE ( 'NONE', #27282, #46306 ) ;
#45124=EDGE_CURVE ( 'NONE', #83062, #34693, #87895, .T. ) ;
#45127=CARTESIAN_POINT ( 'NONE',  ( 69.60148758828984228, 0.4999999999999958922, -9.500000000000000000 ) ) ;
#45131=VECTOR ( 'NONE', #12611, 1000.000000000000000 ) ;
#45168=EDGE_CURVE ( 'NONE', #42904, #18090, #86351, .T. ) ;
#45183=DIRECTION ( 'NONE',  ( -0.000000000000000000, -0.000000000000000000, -1.000000000000000000 ) ) ;
#45194=CARTESIAN_POINT ( 'NONE',  ( 12.26500600480481040, 44.99999999999999289, 0.000000000000000000 ) ) ;
#45197=CARTESIAN_POINT ( 'NONE',  ( 67.06412365047464164, 26.99999999999998224, 9.500000000000000000 ) ) ;
#45224=FACE_OUTER_BOUND ( 'NONE', #20830, .T. ) ;
#45276=CARTESIAN_POINT ( 'NONE',  ( 17.41414817163570916, 33.99863903001855903, 9.761180582272331208 ) ) ;
#45316=DIRECTION ( 'NONE',  ( 0.000000000000000000, 0.000000000000000000, 1.000000000000000000 ) ) ;
#45361=AXIS2_PLACEMENT_3D ( 'NONE', #73619, #12138, #95647 ) ;
#45381=DIRECTION ( 'NONE',  ( -1.000000000000000000, 0.000000000000000000, 0.000000000000000000 ) ) ;
#45419=CARTESIAN_POINT ( 'NONE',  ( -2.253458813454140675, 12.77999999999999936, 9.500000000000000000 ) ) ;
#45490=EDGE_CURVE ( 'NONE', #94289, #53120, #29865, .T. ) ;
#45534=EDGE_CURVE ( 'NONE', #47321, #86750, #78346, .T. ) ;
#45570=AXIS2_PLACEMENT_3D ( 'NONE', #42260, #43228, #58212 ) ;
#45580=DIRECTION ( 'NONE',  ( 1.000000000000000000, -8.673617379884027583E-16, 0.000000000000000000 ) ) ;
#45738=ADVANCED_FACE ( 'NONE', ( #91363 ), #77830, .F. ) ;
#45789=ORIENTED_EDGE ( 'NONE', *, *, #86386, .T. ) ;
#45809=AXIS2_PLACEMENT_3D ( 'NONE', #25920, #47429, #32424 ) ;
#45837=( LENGTH_UNIT ( ) NAMED_UNIT ( * ) SI_UNIT ( .MILLI., .METRE. ) );
#45903=VERTEX_POINT ( 'NONE', #86330 ) ;
#45908=VERTEX_POINT ( 'NONE', #80792 ) ;
#45947=FACE_OUTER_BOUND ( 'NONE', #14689, .T. ) ;
#46000=DIRECTION ( 'NONE',  ( -5.818595309480553908E-17, -1.000000000000000000, -0.000000000000000000 ) ) ;
#46165=AXIS2_PLACEMENT_3D ( 'NONE', #63254, #10274, #1806 ) ;
#46169=VERTEX_POINT ( 'NONE', #67270 ) ;
#46181=EDGE_CURVE ( 'NONE', #20106, #20819, #35279, .T. ) ;
#46298=CARTESIAN_POINT ( 'NONE',  ( 12.26500600480481040, 44.99999999999999289, 0.000000000000000000 ) ) ;
#46306=VECTOR ( 'NONE', #81278, 1000.000000000000000 ) ;
#46341=CARTESIAN_POINT ( 'NONE',  ( 64.56412365047462742, 13.99999999999999467, 9.500000000000000000 ) ) ;
#46403=AXIS2_PLACEMENT_3D ( 'NONE', #23622, #84602, #16101 ) ;
#46502=ORIENTED_EDGE ( 'NONE', *, *, #12686, .F. ) ;
#46514=DIRECTION ( 'NONE',  ( -1.000000000000000000, 0.000000000000000000, 0.000000000000000000 ) ) ;
#46532=ADVANCED_FACE ( 'NONE', ( #43042 ), #57050, .T. ) ;
#46547=EDGE_LOOP ( 'NONE', ( #81523, #65078, #76172, #21924 ) ) ;
#46551=ORIENTED_EDGE ( 'NONE', *, *, #33872, .T. ) ;
#46560=VERTEX_POINT ( 'NONE', #34042 ) ;
#46568=AXIS2_PLACEMENT_3D ( 'NONE', #92095, #76107, #60106 ) ;
#46608=DIRECTION ( 'NONE',  ( -1.000000000000000000, 0.000000000000000000, 0.000000000000000000 ) ) ;
#46691=DIRECTION ( 'NONE',  ( -1.000000000000000000, 0.000000000000000000, -0.000000000000000000 ) ) ;
#46743=DIRECTION ( 'NONE',  ( 0.000000000000000000, -1.000000000000000000, 0.000000000000000000 ) ) ;
#46751=AXIS2_PLACEMENT_3D ( 'NONE', #57971, #88477, #4506 ) ;
#46779=CARTESIAN_POINT ( 'NONE',  ( 32.56412365047463453, 14.00000000000001066, -9.500000000000000000 ) ) ;
#46782=SPHERICAL_SURFACE ( 'NONE', #46165, 0.5000000000000000000 ) ;
#46803=PRESENTATION_STYLE_ASSIGNMENT (( #67846 ) ) ;
#46816=CARTESIAN_POINT ( 'NONE',  ( 0.000000000000000000, 0.5000000000000000000, -10.00000000000000000 ) ) ;
#46856=EDGE_CURVE ( 'NONE', #44442, #61653, #27370, .T. ) ;
#46966=LINE ( 'NONE', #54467, #215 ) ;
#46988=DIRECTION ( 'NONE',  ( -1.000000000000000000, 0.000000000000000000, 0.000000000000000000 ) ) ;
#47098=AXIS2_PLACEMENT_3D ( 'NONE', #85741, #53759, #47730 ) ;
#47102=ORIENTED_EDGE ( 'NONE', *, *, #32000, .F. ) ;
#47130=ORIENTED_EDGE ( 'NONE', *, *, #10761, .T. ) ;
#47132=ORIENTED_EDGE ( 'NONE', *, *, #44628, .T. ) ;
#47176=DIRECTION ( 'NONE',  ( -0.9848077530122086864, -0.1736481776669272781, 0.000000000000000000 ) ) ;
#47221=AXIS2_PLACEMENT_3D ( 'NONE', #36749, #91209, #8223 ) ;
#47242=ORIENTED_EDGE ( 'NONE', *, *, #90792, .T. ) ;
#47321=VERTEX_POINT ( 'NONE', #42352 ) ;
#47350=VECTOR ( 'NONE', #33037, 1000.000000000000000 ) ;
#47375=ORIENTED_EDGE ( 'NONE', *, *, #33872, .F. ) ;
#47429=DIRECTION ( 'NONE',  ( 0.000000000000000000, 0.000000000000000000, 1.000000000000000000 ) ) ;
#47471=ORIENTED_EDGE ( 'NONE', *, *, #39878, .T. ) ;
#47496=FACE_OUTER_BOUND ( 'NONE', #86713, .T. ) ;
#47516=VERTEX_POINT ( 'NONE', #14324 ) ;
#47577=CARTESIAN_POINT ( 'NONE',  ( 32.06412365047463453, 26.99999999999998224, 10.00000000000000000 ) ) ;
#47634=EDGE_CURVE ( 'NONE', #42131, #44141, #85772, .T. ) ;
#47685=DIRECTION ( 'NONE',  ( -0.000000000000000000, -0.000000000000000000, -1.000000000000000000 ) ) ;
#47730=DIRECTION ( 'NONE',  ( -1.000000000000000000, 0.000000000000000000, 0.000000000000000000 ) ) ;
#47768=FACE_OUTER_BOUND ( 'NONE', #11498, .T. ) ;
#47801=DIRECTION ( 'NONE',  ( 1.000000000000000000, -5.818595309480553908E-17, 0.000000000000000000 ) ) ;
#47864=EDGE_LOOP ( 'NONE', ( #91223, #85403 ) ) ;
#47884=VECTOR ( 'NONE', #376, 1000.000000000000000 ) ;
#47917=ADVANCED_FACE ( 'NONE', ( #35102 ), #71162, .T. ) ;
#47919=CARTESIAN_POINT ( 'NONE',  ( 17.85999999999999588, 33.98752635800203592, -10.00000000000000000 ) ) ;
#47963=AXIS2_PLACEMENT_3D ( 'NONE', #83226, #53707, #67239 ) ;
#47966=ORIENTED_EDGE ( 'NONE', *, *, #51780, .T. ) ;
#48000=VERTEX_POINT ( 'NONE', #97623 ) ;
#48019=VERTEX_POINT ( 'NONE', #66603 ) ;
#48100=EDGE_CURVE ( 'NONE', #47321, #66421, #28100, .T. ) ;
#48172=PLANE ( 'NONE',  #72358 ) ;
#48200=CARTESIAN_POINT ( 'NONE',  ( 17.85999999999999943, 37.99999999999997868, -10.00000000000000000 ) ) ;
#48205=ADVANCED_FACE ( 'NONE', ( #37597 ), #60074, .F. ) ;
#48207=AXIS2_PLACEMENT_3D ( 'NONE', #41852, #10853, #19334 ) ;
#48227=ORIENTED_EDGE ( 'NONE', *, *, #32000, .T. ) ;
#48228=LINE ( 'NONE', #40250, #74614 ) ;
#48278=VECTOR ( 'NONE', #9273, 1000.000000000000000 ) ;
#48296=CARTESIAN_POINT ( 'NONE',  ( 34.56412365047464874, 11.49999999999999645, -10.00000000000000000 ) ) ;
#48311=AXIS2_PLACEMENT_3D ( 'NONE', #91930, #23457, #79387 ) ;
#48360=VECTOR ( 'NONE', #35874, 1000.000000000000000 ) ;
#48444=ORIENTED_EDGE ( 'NONE', *, *, #13039, .T. ) ;
#48543=CARTESIAN_POINT ( 'NONE',  ( 64.56412365047462742, 13.99999999999999467, -9.500000000000000000 ) ) ;
#48607=VECTOR ( 'NONE', #46743, 1000.000000000000000 ) ;
#48678=CARTESIAN_POINT ( 'NONE',  ( 17.35999999999999943, 33.99999999999997158, 10.00000000000000000 ) ) ;
#48784=CARTESIAN_POINT ( 'NONE',  ( -0.2838433074297238012, 13.12729635533385597, 10.00000000000000000 ) ) ;
#48821=DIRECTION ( 'NONE',  ( 0.9943711317468826305, 0.1059530667249613811, 0.000000000000000000 ) ) ;
#48825=CARTESIAN_POINT ( 'NONE',  ( 34.56412365047463453, 13.99999999999999645, -10.00000000000000000 ) ) ;
#48862=DIRECTION ( 'NONE',  ( 0.000000000000000000, 0.000000000000000000, 1.000000000000000000 ) ) ;
#48897=CARTESIAN_POINT ( 'NONE',  ( 66.76470751278411342, 40.99999999999997868, 9.500000000000000000 ) ) ;
#49000=VECTOR ( 'NONE', #93527, 1000.000000000000000 ) ;
#49005=CIRCLE ( 'NONE', #7496, 0.5000000000000004441 ) ;
#49144=AXIS2_PLACEMENT_3D ( 'NONE', #17206, #88014, #9193 ) ;
#49151=DIRECTION ( 'NONE',  ( -1.000000000000000000, 0.000000000000000000, 0.000000000000000000 ) ) ;
#49164=FACE_OUTER_BOUND ( 'NONE', #7805, .T. ) ;
#49251=CYLINDRICAL_SURFACE ( 'NONE', #28146, 1.999999999999996669 ) ;
#49284=EDGE_LOOP ( 'NONE', ( #47471, #40254, #51689, #83408, #51106, #31274 ) ) ;
#49323=ORIENTED_EDGE ( 'NONE', *, *, #7735, .T. ) ;
#49325=ADVANCED_FACE ( 'NONE', ( #26890 ), #14839, .T. ) ;
#49396=CARTESIAN_POINT ( 'NONE',  ( 17.35999999999999588, 33.99999999999997868, -9.632054252037207220 ) ) ;
#49398=DIRECTION ( 'NONE',  ( -0.000000000000000000, -0.000000000000000000, 1.000000000000000000 ) ) ;
#49472=ORIENTED_EDGE ( 'NONE', *, *, #5431, .F. ) ;
#49477=EDGE_LOOP ( 'NONE', ( #17601, #23439, #18355, #38109, #83162 ) ) ;
#49498=CIRCLE ( 'NONE', #28735, 1.499999999999996669 ) ;
#49558=EDGE_CURVE ( 'NONE', #93263, #44802, #34875, .T. ) ;
#49561=CARTESIAN_POINT ( 'NONE',  ( -27.43587634952537968, 22.49999999999998934, 10.00000000000000000 ) ) ;
#49567=DIRECTION ( 'NONE',  ( 0.000000000000000000, 0.000000000000000000, -1.000000000000000000 ) ) ;
#49570=AXIS2_PLACEMENT_3D ( 'NONE', #63930, #71942, #33921 ) ;
#49611=VERTEX_POINT ( 'NONE', #61813 ) ;
#49621=CIRCLE ( 'NONE', #6535, 2.500000000000002220 ) ;
#49668=AXIS2_PLACEMENT_3D ( 'NONE', #46341, #8343, #1361 ) ;
#49678=EDGE_CURVE ( 'NONE', #22113, #28657, #16470, .T. ) ;
#49689=CARTESIAN_POINT ( 'NONE',  ( 0.4195498155886417946, 0.4999999999999971689, -9.500000000000000000 ) ) ;
#49875=CIRCLE ( 'NONE', #46751, 0.5000000000000004441 ) ;
#49887=DIRECTION ( 'NONE',  ( -0.000000000000000000, -0.000000000000000000, -1.000000000000000000 ) ) ;
#49890=EDGE_CURVE ( 'NONE', #35983, #44442, #4299, .T. ) ;
#49892=VERTEX_POINT ( 'NONE', #5288 ) ;
#50006=ORIENTED_EDGE ( 'NONE', *, *, #57583, .T. ) ;
#50079=ORIENTED_EDGE ( 'NONE', *, *, #31963, .F. ) ;
#50094=ORIENTED_EDGE ( 'NONE', *, *, #72602, .F. ) ;
#50102=DIRECTION ( 'NONE',  ( 6.938893903907221278E-15, 1.000000000000000000, 0.000000000000000000 ) ) ;
#50126=AXIS2_PLACEMENT_3D ( 'NONE', #86222, #76744, #31729 ) ;
#50170=ORIENTED_EDGE ( 'NONE', *, *, #21940, .F. ) ;
#50172=DIRECTION ( 'NONE',  ( -1.000000000000000000, 0.000000000000000000, 0.000000000000000000 ) ) ;
#50228=FACE_OUTER_BOUND ( 'NONE', #11406, .T. ) ;
#50298=CARTESIAN_POINT ( 'NONE',  ( 31.00000000000000000, -1.803764545938971194E-15, 7.000000000000000000 ) ) ;
#50356=DIRECTION ( 'NONE',  ( 1.000000000000000000, 0.000000000000000000, 0.000000000000000000 ) ) ;
#50394=EDGE_LOOP ( 'NONE', ( #93264, #74581, #76260, #27939 ) ) ;
#50414=AXIS2_PLACEMENT_3D ( 'NONE', #28994, #44000, #98533 ) ;
#50458=EDGE_CURVE ( 'NONE', #77048, #65600, #59951, .T. ) ;
#50461=EDGE_CURVE ( 'NONE', #87279, #49892, #24233, .T. ) ;
#50481=AXIS2_PLACEMENT_3D ( 'NONE', #40306, #70315, #31795 ) ;
#50519=LINE ( 'NONE', #13006, #24159 ) ;
#50598=FILL_AREA_STYLE ('',( #11122 ) ) ;
#50616=ORIENTED_EDGE ( 'NONE', *, *, #50458, .F. ) ;
#50691=LINE ( 'NONE', #66170, #82694 ) ;
#50694=VERTEX_POINT ( 'NONE', #88644 ) ;
#50721=AXIS2_PLACEMENT_3D ( 'NONE', #38844, #6862, #860 ) ;
#50729=EDGE_CURVE ( 'NONE', #35322, #46560, #66134, .T. ) ;
#50736=DIRECTION ( 'NONE',  ( -0.000000000000000000, -0.000000000000000000, -1.000000000000000000 ) ) ;
#50788=DIRECTION ( 'NONE',  ( -0.000000000000000000, -1.000000000000000000, -0.000000000000000000 ) ) ;
#50813=VERTEX_POINT ( 'NONE', #13139 ) ;
#50937=LINE ( 'NONE', #51431, #4534 ) ;
#51044=CIRCLE ( 'NONE', #44621, 0.5000000000000004441 ) ;
#51100=DIRECTION ( 'NONE',  ( 1.000000000000000000, 0.000000000000000000, 0.000000000000000000 ) ) ;
#51106=ORIENTED_EDGE ( 'NONE', *, *, #31963, .T. ) ;
#51115=LINE ( 'NONE', #81603, #2603 ) ;
#51134=CARTESIAN_POINT ( 'NONE',  ( 32.06412365047463453, 14.00000000000001421, -9.500000000000000000 ) ) ;
#51145=EDGE_CURVE ( 'NONE', #20172, #35060, #87135, .T. ) ;
#51163=AXIS2_PLACEMENT_3D ( 'NONE', #90181, #45183, #60672 ) ;
#51196=CIRCLE ( 'NONE', #63950, 0.5000000000000004441 ) ;
#51227=CARTESIAN_POINT ( 'NONE',  ( 69.60148758828984228, -4.049828892140921146E-15, 10.00000000000000000 ) ) ;
#51286=ORIENTED_EDGE ( 'NONE', *, *, #56268, .T. ) ;
#51431=CARTESIAN_POINT ( 'NONE',  ( 32.56412365047463453, 26.99999999999998224, -9.500000000000000000 ) ) ;
#51481=FACE_BOUND ( 'NONE', #95591, .T. ) ;
#51543=FACE_OUTER_BOUND ( 'NONE', #57009, .T. ) ;
#51546=CARTESIAN_POINT ( 'NONE',  ( -4.182615635448454938, 26.60017725333986149, 9.500000000000000000 ) ) ;
#51563=CARTESIAN_POINT ( 'NONE',  ( 38.04706783004212411, -2.213315012455880539E-15, -7.000000000000000000 ) ) ;
#51589=( NAMED_UNIT ( * ) PLANE_ANGLE_UNIT ( ) SI_UNIT ( $, .RADIAN. ) );
#51647=TOROIDAL_SURFACE ( 'NONE', #24470, 20.49999999999999645, 0.5000000000000000000 ) ;
#51661=AXIS2_PLACEMENT_3D ( 'NONE', #78275, #31782, #24314 ) ;
#51689=ORIENTED_EDGE ( 'NONE', *, *, #65283, .F. ) ;
#51699=EDGE_LOOP ( 'NONE', ( #19189, #59580, #66175, #25281, #87607, #59993, #54995, #88552 ) ) ;
#51757=VERTEX_POINT ( 'NONE', #74781 ) ;
#51780=EDGE_CURVE ( 'NONE', #89049, #87399, #6290, .T. ) ;
#51806=EDGE_LOOP ( 'NONE', ( #93593, #68672, #81054, #64474 ) ) ;
#51848=COLOUR_RGB ( '', 0.72549020, 0.75294118, 0.79215686) ;
#51863=CARTESIAN_POINT ( 'NONE',  ( 64.56412365047461321, -3.756725070333740926E-15, 0.000000000000000000 ) ) ;
#51877=AXIS2_PLACEMENT_3D ( 'NONE', #16346, #92821, #76352 ) ;
#51880=DIRECTION ( 'NONE',  ( 1.000000000000000000, 1.636349903325072848E-16, 0.000000000000000000 ) ) ;
#51887=EDGE_LOOP ( 'NONE', ( #62548, #34307, #79129, #52677 ) ) ;
#51915=EDGE_CURVE ( 'NONE', #44442, #66734, #80593, .T. ) ;
#52077=ORIENTED_EDGE ( 'NONE', *, *, #10978, .T. ) ;
#52101=AXIS2_PLACEMENT_3D ( 'NONE', #77577, #25102, #16107 ) ;
#52200=CARTESIAN_POINT ( 'NONE',  ( 34.56412365047464874, 11.49999999999999645, 10.00000000000000000 ) ) ;
#52203=AXIS2_PLACEMENT_3D ( 'NONE', #35218, #50736, #73713 ) ;
#52208=ORIENTED_EDGE ( 'NONE', *, *, #65393, .F. ) ;
#52238=CARTESIAN_POINT ( 'NONE',  ( 64.56412365047461321, 11.99999999999999467, -7.000000000000000888 ) ) ;
#52291=VECTOR ( 'NONE', #68849, 1000.000000000000000 ) ;
#52323=LINE ( 'NONE', #76792, #442 ) ;
#52345=PLANE ( 'NONE',  #39198 ) ;
#52382=DIRECTION ( 'NONE',  ( 0.000000000000000000, 0.000000000000000000, -1.000000000000000000 ) ) ;
#52521=CARTESIAN_POINT ( 'NONE',  ( 64.56412365047461321, 29.50000000000000000, 9.500000000000000000 ) ) ;
#52581=DIRECTION ( 'NONE',  ( -0.000000000000000000, -0.000000000000000000, 1.000000000000000000 ) ) ;
#52677=ORIENTED_EDGE ( 'NONE', *, *, #16297, .F. ) ;
#52688=CARTESIAN_POINT ( 'NONE',  ( -0.2838433074297238012, 13.12729635533385597, 9.500000000000000000 ) ) ;
#52776=EDGE_LOOP ( 'NONE', ( #50006, #32352, #83662, #55928 ) ) ;
#52826=CIRCLE ( 'NONE', #87942, 4.000000000000003553 ) ;
#52833=CARTESIAN_POINT ( 'NONE',  ( 27.50000000000000355, 35.99999999999997158, -7.000000000000000000 ) ) ;
#52844=DIRECTION ( 'NONE',  ( 1.000000000000000000, 0.000000000000000000, 0.000000000000000000 ) ) ;
#52850=ORIENTED_EDGE ( 'NONE', *, *, #82319, .F. ) ;
#52884=CARTESIAN_POINT ( 'NONE',  ( 67.06412365047464164, 26.99999999999998224, 9.500000000000000000 ) ) ;
#52892=AXIS2_PLACEMENT_3D ( 'NONE', #38354, #68847, #15850 ) ;
#52990=VECTOR ( 'NONE', #6624, 1000.000000000000000 ) ;
#52996=DIRECTION ( 'NONE',  ( 0.000000000000000000, 0.000000000000000000, 1.000000000000000000 ) ) ;
#53066=CIRCLE ( 'NONE', #14775, 0.5000000000000004441 ) ;
#53106=CARTESIAN_POINT ( 'NONE',  ( -1.761054936948036165, 12.86682408883346440, -10.00000000000000000 ) ) ;
#53109=ADVANCED_FACE ( 'NONE', ( #21867 ), #52345, .T. ) ;
#53118=LINE ( 'NONE', #72774, #92622 ) ;
#53120=VERTEX_POINT ( 'NONE', #52833 ) ;
#53129=DIRECTION ( 'NONE',  ( -5.818595309480553908E-17, -1.000000000000000000, -0.000000000000000000 ) ) ;
#53155=VERTEX_POINT ( 'NONE', #82842 ) ;
#53197=CARTESIAN_POINT ( 'NONE',  ( 34.56412365047463453, 13.99999999999999645, 10.00000000000000000 ) ) ;
#53206=LINE ( 'NONE', #82715, #87445 ) ;
#53288=ORIENTED_EDGE ( 'NONE', *, *, #37520, .F. ) ;
#53352=ORIENTED_EDGE ( 'NONE', *, *, #95101, .T. ) ;
#53387=DIRECTION ( 'NONE',  ( -0.000000000000000000, -0.000000000000000000, -1.000000000000000000 ) ) ;
#53484=MECHANICAL_DESIGN_GEOMETRIC_PRESENTATION_REPRESENTATION('',(#23104),#82176);
#53598=DIRECTION ( 'NONE',  ( 0.000000000000000000, 0.000000000000000000, 1.000000000000000000 ) ) ;
#53627=CIRCLE ( 'NONE', #10519, 100.0000000000000000 ) ;
#53707=DIRECTION ( 'NONE',  ( -0.000000000000000000, -0.000000000000000000, -1.000000000000000000 ) ) ;
#53719=SHAPE_REPRESENTATION ( '1.1 Cage', ( #27931 ), #96613 ) ;
#53735=EDGE_LOOP ( 'NONE', ( #21815, #94980, #96396, #6358 ) ) ;
#53759=DIRECTION ( 'NONE',  ( -0.000000000000000000, -0.000000000000000000, -1.000000000000000000 ) ) ;
#53789=CARTESIAN_POINT ( 'NONE',  ( 64.56412365047461321, 44.99999999999998579, 7.000000000000000000 ) ) ;
#53949=CARTESIAN_POINT ( 'NONE',  ( 5.000000000000002665, 44.99999999999999289, 0.000000000000000000 ) ) ;
#53983=CIRCLE ( 'NONE', #57178, 20.00000000000000000 ) ;
#54008=EDGE_LOOP ( 'NONE', ( #41152, #18217, #52850, #38568 ) ) ;
#54155=DIRECTION ( 'NONE',  ( -1.000000000000000000, 0.000000000000000000, 0.000000000000000000 ) ) ;
#54181=ADVANCED_FACE ( 'NONE', ( #3176 ), #33641, .F. ) ;
#54190=CARTESIAN_POINT ( 'NONE',  ( 2.618367889266248100E-15, 44.99999999999999289, -7.000000000000000000 ) ) ;
#54236=DIRECTION ( 'NONE',  ( 0.000000000000000000, 1.000000000000000000, 0.000000000000000000 ) ) ;
#54423=CARTESIAN_POINT ( 'NONE',  ( 66.76470751278411342, 44.99999999999998579, -9.500000000000000000 ) ) ;
#54428=CARTESIAN_POINT ( 'NONE',  ( 70.08911253270098030, 0.3894472361808988259, -9.500000000000000000 ) ) ;
#54452=CARTESIAN_POINT ( 'NONE',  ( 32.26500600480481040, -1.876920803484231371E-15, 0.000000000000000000 ) ) ;
#54467=CARTESIAN_POINT ( 'NONE',  ( 64.56412365047461321, 44.99999999999998579, -7.000000000000000000 ) ) ;
#54506=ORIENTED_EDGE ( 'NONE', *, *, #624, .F. ) ;
#54554=ORIENTED_EDGE ( 'NONE', *, *, #71268, .F. ) ;
#54575=CARTESIAN_POINT ( 'NONE',  ( 67.06412365047464164, 14.00000000000001243, 10.00000000000000000 ) ) ;
#54596=FACE_OUTER_BOUND ( 'NONE', #65561, .T. ) ;
#54653=EDGE_CURVE ( 'NONE', #66421, #85266, #80799, .T. ) ;
#54700=DIRECTION ( 'NONE',  ( -1.000000000000000000, -1.636349903325072848E-16, 0.000000000000000000 ) ) ;
#54745=EDGE_CURVE ( 'NONE', #40893, #3546, #90415, .T. ) ;
#54813=CYLINDRICAL_SURFACE ( 'NONE', #17982, 1.500000000000001332 ) ;
#54844=AXIS2_PLACEMENT_3D ( 'NONE', #89590, #27104, #27602 ) ;
#54855=EDGE_CURVE ( 'NONE', #44141, #10785, #5792, .T. ) ;
#54984=DIRECTION ( 'NONE',  ( -1.000000000000000000, 0.000000000000000000, -0.000000000000000000 ) ) ;
#54989=EDGE_CURVE ( 'NONE', #61653, #11334, #85906, .T. ) ;
#54995=ORIENTED_EDGE ( 'NONE', *, *, #88394, .T. ) ;
#55055=DIRECTION ( 'NONE',  ( -0.000000000000000000, -0.000000000000000000, -1.000000000000000000 ) ) ;
#55111=CIRCLE ( 'NONE', #67911, 19.99999999999999645 ) ;
#55127=ORIENTED_EDGE ( 'NONE', *, *, #44146, .T. ) ;
#55136=EDGE_CURVE ( 'NONE', #38557, #63645, #94696, .T. ) ;
#55138=VECTOR ( 'NONE', #86525, 1000.000000000000000 ) ;
#55148=ORIENTED_EDGE ( 'NONE', *, *, #8493, .F. ) ;
#55254=VERTEX_POINT ( 'NONE', #44135 ) ;
#55262=ADVANCED_FACE ( 'NONE', ( #97671 ), #81646, .T. ) ;
#55310=STYLED_ITEM ( 'NONE', ( #41641 ), #41283 ) ;
#55367=AXIS2_PLACEMENT_3D ( 'NONE', #13737, #73238, #96265 ) ;
#55436=CYLINDRICAL_SURFACE ( 'NONE', #9111, 100.0000000000000000 ) ;
#55479=DIRECTION ( 'NONE',  ( 0.9848077530122086864, 0.1736481776669272503, -0.000000000000000000 ) ) ;
#55541=ORIENTED_EDGE ( 'NONE', *, *, #31881, .F. ) ;
#55551=ORIENTED_EDGE ( 'NONE', *, *, #91196, .F. ) ;
#55558=VECTOR ( 'NONE', #79090, 1000.000000000000000 ) ;
#55660=CARTESIAN_POINT ( 'NONE',  ( 0.000000000000000000, 0.000000000000000000, -9.500000000000000000 ) ) ;
#55693=DIRECTION ( 'NONE',  ( -0.000000000000000000, -0.000000000000000000, -1.000000000000000000 ) ) ;
#55729=ORIENTED_EDGE ( 'NONE', *, *, #78016, .F. ) ;
#55909=ORIENTED_EDGE ( 'NONE', *, *, #1891, .T. ) ;
#55928=ORIENTED_EDGE ( 'NONE', *, *, #44112, .T. ) ;
#56032=DIRECTION ( 'NONE',  ( -1.000000000000000000, 0.000000000000000000, 0.000000000000000000 ) ) ;
#56146=CIRCLE ( 'NONE', #48207, 20.49999999999999645 ) ;
#56156=ORIENTED_EDGE ( 'NONE', *, *, #97151, .F. ) ;
#56157=CARTESIAN_POINT ( 'NONE',  ( 34.56412365047464874, 28.99999999999999645, 7.000000000000000000 ) ) ;
#56169=DIRECTION ( 'NONE',  ( 0.000000000000000000, -1.000000000000000000, 0.000000000000000000 ) ) ;
#56218=VERTEX_POINT ( 'NONE', #32531 ) ;
#56240=EDGE_LOOP ( 'NONE', ( #6709, #4391, #42870, #89939, #42970, #85281, #9369, #67579, #27832, #28092 ) ) ;
#56268=EDGE_CURVE ( 'NONE', #30184, #28589, #17553, .T. ) ;
#56278=PLANE ( 'NONE',  #51661 ) ;
#56279=DIRECTION ( 'NONE',  ( -0.000000000000000000, -0.000000000000000000, 1.000000000000000000 ) ) ;
#56286=AXIS2_PLACEMENT_3D ( 'NONE', #74886, #30360, #52382 ) ;
#56297=AXIS2_PLACEMENT_3D ( 'NONE', #97387, #4901, #89859 ) ;
#56307=DIRECTION ( 'NONE',  ( -1.000000000000000000, 0.000000000000000000, -0.000000000000000000 ) ) ;
#56388=EDGE_LOOP ( 'NONE', ( #6010, #78370, #77059, #77253 ) ) ;
#56390=EDGE_CURVE ( 'NONE', #63645, #51757, #90546, .T. ) ;
#56410=EDGE_LOOP ( 'NONE', ( #60960, #23426, #60579, #59085 ) ) ;
#56503=AXIS2_PLACEMENT_3D ( 'NONE', #31684, #32670, #47176 ) ;
#56516=VERTEX_POINT ( 'NONE', #74978 ) ;
#56529=ORIENTED_EDGE ( 'NONE', *, *, #7710, .T. ) ;
#56547=DIRECTION ( 'NONE',  ( -0.000000000000000000, -0.000000000000000000, -1.000000000000000000 ) ) ;
#56556=CARTESIAN_POINT ( 'NONE',  ( 38.04706783004212411, 44.99999999999999289, -7.000000000000000000 ) ) ;
#56557=CARTESIAN_POINT ( 'NONE',  ( -0.07285406091746288171, 0.4131759111665360140, 9.500000000000000000 ) ) ;
#56558=EDGE_CURVE ( 'NONE', #65600, #60520, #88913, .T. ) ;
#56614=CARTESIAN_POINT ( 'NONE',  ( -1.761054936948033278, 12.86682408883346440, 9.500000000000000000 ) ) ;
#56717=ORIENTED_EDGE ( 'NONE', *, *, #49890, .T. ) ;
#56740=VECTOR ( 'NONE', #34651, 1000.000000000000000 ) ;
#56754=CARTESIAN_POINT ( 'NONE',  ( 26.00000000000000355, 35.99999999999997158, -10.00000000000000000 ) ) ;
#56766=CIRCLE ( 'NONE', #50414, 0.4999999999999998335 ) ;
#56784=ORIENTED_EDGE ( 'NONE', *, *, #3766, .T. ) ;
#56904=AXIS2_PLACEMENT_3D ( 'NONE', #42127, #27097, #64593 ) ;
#57009=EDGE_LOOP ( 'NONE', ( #52077, #28150, #96810, #88592 ) ) ;
#57050=CYLINDRICAL_SURFACE ( 'NONE', #59284, 0.5000000000000004441 ) ;
#57071=ORIENTED_EDGE ( 'NONE', *, *, #10978, .F. ) ;
#57178=AXIS2_PLACEMENT_3D ( 'NONE', #18973, #26456, #79957 ) ;
#57225=EDGE_CURVE ( 'NONE', #20106, #62619, #98734, .T. ) ;
#57239=PLANE ( 'NONE',  #38897 ) ;
#57378=EDGE_CURVE ( 'NONE', #84180, #1194, #2681, .T. ) ;
#57409=CARTESIAN_POINT ( 'NONE',  ( 70.08911253270099451, 0.3894472361808953842, 10.00000000000000000 ) ) ;
#57472=VERTEX_POINT ( 'NONE', #39188 ) ;
#57506=TOROIDAL_SURFACE ( 'NONE', #97507, 1.499999999999996669, 0.5000000000000000000 ) ;
#57583=EDGE_CURVE ( 'NONE', #1778, #38557, #85661, .T. ) ;
#57668=VECTOR ( 'NONE', #83357, 1000.000000000000000 ) ;
#57955=EDGE_CURVE ( 'NONE', #34693, #16030, #31193, .T. ) ;
#57971=CARTESIAN_POINT ( 'NONE',  ( 66.76470751278411342, 44.49999999999998579, 9.500000000000000000 ) ) ;
#58065=EDGE_LOOP ( 'NONE', ( #92486, #35786 ) ) ;
#58135=EDGE_CURVE ( 'NONE', #28589, #56516, #87478, .T. ) ;
#58156=DIRECTION ( 'NONE',  ( 0.000000000000000000, 0.000000000000000000, 1.000000000000000000 ) ) ;
#58212=DIRECTION ( 'NONE',  ( -1.000000000000000000, 0.000000000000000000, 0.000000000000000000 ) ) ;
#58232=CARTESIAN_POINT ( 'NONE',  ( 70.68973184038034674, 41.77083333333331439, 9.500000000000000000 ) ) ;
#58296=EDGE_CURVE ( 'NONE', #77048, #46169, #10833, .T. ) ;
#58327=DIRECTION ( 'NONE',  ( -1.000000000000000000, 0.000000000000000000, 0.000000000000000000 ) ) ;
#58361=DIRECTION ( 'NONE',  ( -0.000000000000000000, -1.000000000000000000, -0.000000000000000000 ) ) ;
#58369=CARTESIAN_POINT ( 'NONE',  ( 24.35999999999999233, 44.49999999999997868, -9.500000000000000000 ) ) ;
#58413=EDGE_CURVE ( 'NONE', #56516, #55254, #7636, .T. ) ;
#58490=DIRECTION ( 'NONE',  ( -1.000000000000000000, 0.000000000000000000, 0.000000000000000000 ) ) ;
#58519=DIRECTION ( 'NONE',  ( 0.000000000000000000, 0.000000000000000000, 1.000000000000000000 ) ) ;
#58572=AXIS2_PLACEMENT_3D ( 'NONE', #88503, #20006, #58490 ) ;
#58579=ORIENTED_EDGE ( 'NONE', *, *, #23968, .F. ) ;
#58594=AXIS2_PLACEMENT_3D ( 'NONE', #91680, #23198, #8666 ) ;
#58624=DIRECTION ( 'NONE',  ( -1.000000000000000000, 0.000000000000000000, 0.000000000000000000 ) ) ;
#58655=DIRECTION ( 'NONE',  ( 1.000000000000000000, 0.000000000000000000, 0.000000000000000000 ) ) ;
#58692=ORIENTED_EDGE ( 'NONE', *, *, #16297, .T. ) ;
#58697=CIRCLE ( 'NONE', #15617, 1.999999999999996669 ) ;
#58748=CARTESIAN_POINT ( 'NONE',  ( 56.78206182523731371, 44.99999999999999289, 0.000000000000000000 ) ) ;
#58780=AXIS2_PLACEMENT_3D ( 'NONE', #84033, #30519, #46514 ) ;
#58817=DIRECTION ( 'NONE',  ( -5.818595309480553908E-17, -1.000000000000000000, -0.000000000000000000 ) ) ;
#58974=CARTESIAN_POINT ( 'NONE',  ( 0.4195498155886339120, 0.5000000000000038858, 9.500000000000000000 ) ) ;
#59014=DIRECTION ( 'NONE',  ( 8.673617379884027583E-16, 1.000000000000000000, 0.000000000000000000 ) ) ;
#59032=AXIS2_PLACEMENT_3D ( 'NONE', #6855, #14868, #32294 ) ;
#59068=ORIENTED_EDGE ( 'NONE', *, *, #57378, .F. ) ;
#59077=CIRCLE ( 'NONE', #6408, 0.5000000000000004441 ) ;
#59081=ORIENTED_EDGE ( 'NONE', *, *, #20098, .F. ) ;
#59085=ORIENTED_EDGE ( 'NONE', *, *, #79251, .T. ) ;
#59181=EDGE_LOOP ( 'NONE', ( #31521, #32286, #79515, #73688 ) ) ;
#59219=EDGE_LOOP ( 'NONE', ( #95355, #50616, #63425, #31395 ) ) ;
#59284=AXIS2_PLACEMENT_3D ( 'NONE', #4069, #81521, #80050 ) ;
#59314=ORIENTED_EDGE ( 'NONE', *, *, #94367, .T. ) ;
#59321=CYLINDRICAL_SURFACE ( 'NONE', #40302, 19.99999999999999645 ) ;
#59335=DIRECTION ( 'NONE',  ( 0.000000000000000000, 0.000000000000000000, 1.000000000000000000 ) ) ;
#59378=CARTESIAN_POINT ( 'NONE',  ( 27.50000000000000355, 35.99999999999997158, -10.00000000000000000 ) ) ;
#59423=VECTOR ( 'NONE', #86604, 1000.000000000000000 ) ;
#59434=EDGE_CURVE ( 'NONE', #10785, #11195, #29756, .T. ) ;
#59468=DIRECTION ( 'NONE',  ( -1.000000000000000000, 0.000000000000000000, -0.000000000000000000 ) ) ;
#59520=ORIENTED_EDGE ( 'NONE', *, *, #76323, .F. ) ;
#59524=DIRECTION ( 'NONE',  ( -1.000000000000000000, 2.081668171172166620E-14, 0.000000000000000000 ) ) ;
#59551=ORIENTED_EDGE ( 'NONE', *, *, #65380, .T. ) ;
#59577=DIRECTION ( 'NONE',  ( -1.000000000000000000, 0.000000000000000000, 0.000000000000000000 ) ) ;
#59580=ORIENTED_EDGE ( 'NONE', *, *, #29117, .T. ) ;
#59629=ORIENTED_EDGE ( 'NONE', *, *, #20467, .T. ) ;
#59631=EDGE_CURVE ( 'NONE', #94846, #25948, #86365, .T. ) ;
#59640=CIRCLE ( 'NONE', #18618, 2.500000000000002220 ) ;
#59697=AXIS2_PLACEMENT_3D ( 'NONE', #63164, #47685, #9689 ) ;
#59709=EDGE_CURVE ( 'NONE', #66451, #22113, #38179, .T. ) ;
#59834=ORIENTED_EDGE ( 'NONE', *, *, #97920, .T. ) ;
#59848=CYLINDRICAL_SURFACE ( 'NONE', #10657, 6.999999999999995559 ) ;
#59852=SPHERICAL_SURFACE ( 'NONE', #56297, 0.5000000000000000000 ) ;
#59951=CIRCLE ( 'NONE', #88711, 1.499999999999996669 ) ;
#59972=AXIS2_PLACEMENT_3D ( 'NONE', #51546, #96569, #95570 ) ;
#59993=ORIENTED_EDGE ( 'NONE', *, *, #65393, .T. ) ;
#60074=CYLINDRICAL_SURFACE ( 'NONE', #24328, 2.000000000000001776 ) ;
#60106=DIRECTION ( 'NONE',  ( 1.000000000000000000, -5.818595309480553908E-17, 0.000000000000000000 ) ) ;
#60197=VERTEX_POINT ( 'NONE', #80085 ) ;
#60204=CARTESIAN_POINT ( 'NONE',  ( 66.76470751278411342, 40.99999999999997868, -9.500000000000000000 ) ) ;
#60232=CARTESIAN_POINT ( 'NONE',  ( 64.56412365047461321, 28.99999999999999645, 10.00000000000000000 ) ) ;
#60264=CARTESIAN_POINT ( 'NONE',  ( 17.35999999999999588, 33.99999999999997158, -9.500000000000000000 ) ) ;
#60298=CARTESIAN_POINT ( 'NONE',  ( 24.50000000000000000, 35.99999999999997158, 7.000000000000000888 ) ) ;
#60326=CARTESIAN_POINT ( 'NONE',  ( 24.50000000000000000, 35.99999999999997158, 10.00000000000000000 ) ) ;
#60359=ORIENTED_EDGE ( 'NONE', *, *, #77894, .F. ) ;
#60391=ORIENTED_EDGE ( 'NONE', *, *, #27712, .F. ) ;
#60396=CYLINDRICAL_SURFACE ( 'NONE', #77596, 6.999999999999995559 ) ;
#60443=ORIENTED_EDGE ( 'NONE', *, *, #95101, .F. ) ;
#60520=VERTEX_POINT ( 'NONE', #78501 ) ;
#60579=ORIENTED_EDGE ( 'NONE', *, *, #43446, .F. ) ;
#60597=DIRECTION ( 'NONE',  ( -0.000000000000000000, -0.000000000000000000, -1.000000000000000000 ) ) ;
#60645=AXIS2_PLACEMENT_3D ( 'NONE', #86451, #87419, #70961 ) ;
#60672=DIRECTION ( 'NONE',  ( -1.000000000000000000, 0.000000000000000000, 0.000000000000000000 ) ) ;
#60921=ORIENTED_EDGE ( 'NONE', *, *, #48100, .T. ) ;
#60928=FACE_OUTER_BOUND ( 'NONE', #21842, .T. ) ;
#60958=EDGE_CURVE ( 'NONE', #61160, #92057, #87256, .T. ) ;
#60960=ORIENTED_EDGE ( 'NONE', *, *, #65283, .T. ) ;
#61009=CARTESIAN_POINT ( 'NONE',  ( -1.783843307429720415, 13.12729635533385597, -10.00000000000000000 ) ) ;
#61011=ORIENTED_EDGE ( 'NONE', *, *, #1268, .T. ) ;
#61042=EDGE_LOOP ( 'NONE', ( #10878, #59834, #41561, #71707 ) ) ;
#61054=ORIENTED_EDGE ( 'NONE', *, *, #82507, .F. ) ;
#61080=ORIENTED_EDGE ( 'NONE', *, *, #73156, .T. ) ;
#61097=DIRECTION ( 'NONE',  ( -8.673617379884027583E-16, -1.000000000000000000, 0.000000000000000000 ) ) ;
#61142=ORIENTED_EDGE ( 'NONE', *, *, #26876, .F. ) ;
#61145=VERTEX_POINT ( 'NONE', #244 ) ;
#61160=VERTEX_POINT ( 'NONE', #76217 ) ;
#61170=VECTOR ( 'NONE', #87416, 1000.000000000000000 ) ;
#61382=ORIENTED_EDGE ( 'NONE', *, *, #59709, .F. ) ;
#61420=CYLINDRICAL_SURFACE ( 'NONE', #35543, 2.000000000000001776 ) ;
#61583=DIRECTION ( 'NONE',  ( -0.1736481776669272503, 0.9848077530122086864, 0.000000000000000000 ) ) ;
#61597=CARTESIAN_POINT ( 'NONE',  ( 34.56412365047464874, 28.99999999999999645, -9.500000000000000000 ) ) ;
#61647=AXIS2_PLACEMENT_3D ( 'NONE', #43119, #12131, #42631 ) ;
#61653=VERTEX_POINT ( 'NONE', #40676 ) ;
#61729=DIRECTION ( 'NONE',  ( 1.000000000000000000, -5.782411586589362323E-17, 0.000000000000000000 ) ) ;
#61748=AXIS2_PLACEMENT_3D ( 'NONE', #1353, #32298, #77308 ) ;
#61760=ADVANCED_FACE ( 'NONE', ( #41181 ), #11313, .T. ) ;
#61776=TOROIDAL_SURFACE ( 'NONE', #58572, 99.50000000000000000, 0.5000000000000000000 ) ;
#61813=CARTESIAN_POINT ( 'NONE',  ( 17.35999999999999588, 33.99999999999997158, -7.000000000000000888 ) ) ;
#61827=DIRECTION ( 'NONE',  ( -0.000000000000000000, -0.000000000000000000, 1.000000000000000000 ) ) ;
#61844=DIRECTION ( 'NONE',  ( -0.000000000000000000, -0.000000000000000000, -1.000000000000000000 ) ) ;
#61854=VECTOR ( 'NONE', #77168, 1000.000000000000000 ) ;
#61925=EDGE_CURVE ( 'NONE', #16030, #15047, #49621, .T. ) ;
#61998=CARTESIAN_POINT ( 'NONE',  ( 64.56412365047461321, 11.49999999999999467, -10.00000000000000000 ) ) ;
#62023=VERTEX_POINT ( 'NONE', #64036 ) ;
#62077=DIRECTION ( 'NONE',  ( -1.000000000000000000, -0.000000000000000000, -0.000000000000000000 ) ) ;
#62095=LINE ( 'NONE', #15152, #28231 ) ;
#62116=DIRECTION ( 'NONE',  ( 0.000000000000000000, 0.000000000000000000, 1.000000000000000000 ) ) ;
#62153=VECTOR ( 'NONE', #42883, 1000.000000000000000 ) ;
#62163=VECTOR ( 'NONE', #96917, 1000.000000000000000 ) ;
#62209=CARTESIAN_POINT ( 'NONE',  ( 67.06412365047464164, 14.00000000000000888, -10.00000000000000000 ) ) ;
#62238=ADVANCED_FACE ( 'NONE', ( #39604 ), #74507, .F. ) ;
#62256=ORIENTED_EDGE ( 'NONE', *, *, #13597, .T. ) ;
#62280=VECTOR ( 'NONE', #17284, 1000.000000000000000 ) ;
#62304=CARTESIAN_POINT ( 'NONE',  ( 0.4195498155886495661, 0.4999999999999985012, -9.500000000000000000 ) ) ;
#62309=DIRECTION ( 'NONE',  ( -1.000000000000000000, 0.000000000000000000, 0.000000000000000000 ) ) ;
#62375=DIRECTION ( 'NONE',  ( 1.000000000000000000, 0.000000000000000000, 0.000000000000000000 ) ) ;
#62479=AXIS2_PLACEMENT_3D ( 'NONE', #68505, #46000, #22027 ) ;
#62498=CIRCLE ( 'NONE', #97649, 19.99999999999999645 ) ;
#62546=ADVANCED_FACE ( 'NONE', ( #68011 ), #15022, .F. ) ;
#62548=ORIENTED_EDGE ( 'NONE', *, *, #40534, .T. ) ;
#62571=CARTESIAN_POINT ( 'NONE',  ( 34.56412365047464874, 29.50000000000000000, -9.500000000000000000 ) ) ;
#62619=VERTEX_POINT ( 'NONE', #98033 ) ;
#62626=ORIENTED_EDGE ( 'NONE', *, *, #80132, .T. ) ;
#62640=ORIENTED_EDGE ( 'NONE', *, *, #416, .F. ) ;
#62641=EDGE_CURVE ( 'NONE', #53155, #35322, #8489, .T. ) ;
#62689=VERTEX_POINT ( 'NONE', #15993 ) ;
#62741=AXIS2_PLACEMENT_3D ( 'NONE', #36127, #79667, #20645 ) ;
#62760=EDGE_CURVE ( 'NONE', #62619, #67069, #46966, .T. ) ;
#62764=CARTESIAN_POINT ( 'NONE',  ( 17.35999999999999943, 37.99999999999997868, -9.500000000000000000 ) ) ;
#62935=PLANE ( 'NONE',  #33848 ) ;
#62951=ORIENTED_EDGE ( 'NONE', *, *, #51145, .T. ) ;
#62975=EDGE_CURVE ( 'NONE', #46169, #35983, #35286, .T. ) ;
#63136=TOROIDAL_SURFACE ( 'NONE', #18401, 2.500000000000000888, 0.5000000000000000000 ) ;
#63150=VERTEX_POINT ( 'NONE', #89628 ) ;
#63164=CARTESIAN_POINT ( 'NONE',  ( 64.56412365047462742, 13.99999999999999467, 10.00000000000000000 ) ) ;
#63217=EDGE_CURVE ( 'NONE', #94289, #27691, #41744, .T. ) ;
#63240=ORIENTED_EDGE ( 'NONE', *, *, #35159, .T. ) ;
#63254=CARTESIAN_POINT ( 'NONE',  ( 0.4195498155886317471, 0.5000000000000013323, 9.500000000000000000 ) ) ;
#63270=EDGE_CURVE ( 'NONE', #65600, #63150, #36948, .T. ) ;
#63321=VECTOR ( 'NONE', #22860, 1000.000000000000000 ) ;
#63343=VERTEX_POINT ( 'NONE', #54575 ) ;
#63373=CARTESIAN_POINT ( 'NONE',  ( 24.35999999999999233, 44.49999999999997868, -9.500000000000000000 ) ) ;
#63425=ORIENTED_EDGE ( 'NONE', *, *, #58296, .T. ) ;
#63443=EDGE_CURVE ( 'NONE', #92229, #81201, #76900, .T. ) ;
#63448=EDGE_CURVE ( 'NONE', #63645, #82054, #14644, .T. ) ;
#63493=AXIS2_PLACEMENT_3D ( 'NONE', #62304, #83352, #52844 ) ;
#63571=CARTESIAN_POINT ( 'NONE',  ( -2.283843307429720415, 13.12729635533385597, 10.00000000000000000 ) ) ;
#63641=CARTESIAN_POINT ( 'NONE',  ( 32.06412365047463453, 22.49999999999998934, -9.500000000000000000 ) ) ;
#63645=VERTEX_POINT ( 'NONE', #56557 ) ;
#63647=CARTESIAN_POINT ( 'NONE',  ( -27.43587634952537968, 22.49999999999998934, 9.500000000000000000 ) ) ;
#63734=AXIS2_PLACEMENT_3D ( 'NONE', #79410, #3910, #41918 ) ;
#63841=CIRCLE ( 'NONE', #38321, 6.499999999999995559 ) ;
#63843=ORIENTED_EDGE ( 'NONE', *, *, #7710, .F. ) ;
#63863=CARTESIAN_POINT ( 'NONE',  ( -27.43587634952537968, 22.49999999999998934, 10.00000000000000000 ) ) ;
#63896=CARTESIAN_POINT ( 'NONE',  ( -27.43587634952537968, 22.49999999999998934, 10.00000000000000000 ) ) ;
#63930=CARTESIAN_POINT ( 'NONE',  ( -2.614810775378867191, 35.00346125376525919, -10.00000000000000000 ) ) ;
#63932=FACE_OUTER_BOUND ( 'NONE', #52776, .T. ) ;
#63950=AXIS2_PLACEMENT_3D ( 'NONE', #28102, #11139, #41658 ) ;
#63978=EDGE_LOOP ( 'NONE', ( #25760, #32529, #75481, #94413 ) ) ;
#64006=ORIENTED_EDGE ( 'NONE', *, *, #34653, .F. ) ;
#64020=ORIENTED_EDGE ( 'NONE', *, *, #63270, .T. ) ;
#64036=CARTESIAN_POINT ( 'NONE',  ( 66.56412365047464164, 26.99999999999998224, 9.500000000000000000 ) ) ;
#64129=CARTESIAN_POINT ( 'NONE',  ( 31.00000000000000355, 44.99999999999999289, 7.000000000000000000 ) ) ;
#64203=ORIENTED_EDGE ( 'NONE', *, *, #33404, .T. ) ;
#64222=CYLINDRICAL_SURFACE ( 'NONE', #70304, 1.500000000000001332 ) ;
#64225=CIRCLE ( 'NONE', #21141, 0.5000000000000000000 ) ;
#64320=EDGE_CURVE ( 'NONE', #55254, #23929, #24322, .T. ) ;
#64367=DIRECTION ( 'NONE',  ( 0.000000000000000000, 0.000000000000000000, 1.000000000000000000 ) ) ;
#64390=CARTESIAN_POINT ( 'NONE',  ( 17.41414817163570916, 33.99863903001854482, -9.761180582272329431 ) ) ;
#64405=AXIS2_PLACEMENT_3D ( 'NONE', #70483, #55479, #32956 ) ;
#64461=ADVANCED_FACE ( 'NONE', ( #87236 ), #75400, .T. ) ;
#64470=ORIENTED_EDGE ( 'NONE', *, *, #79044, .F. ) ;
#64474=ORIENTED_EDGE ( 'NONE', *, *, #44628, .F. ) ;
#64584=EDGE_LOOP ( 'NONE', ( #75791, #44738, #43454, #56529 ) ) ;
#64593=DIRECTION ( 'NONE',  ( -1.000000000000000000, 0.000000000000000000, 0.000000000000000000 ) ) ;
#64627=DIRECTION ( 'NONE',  ( -1.000000000000000000, 0.000000000000000000, 0.000000000000000000 ) ) ;
#64659=CARTESIAN_POINT ( 'NONE',  ( 24.35999999999999233, 44.99999999999997158, 9.500000000000000000 ) ) ;
#64682=CARTESIAN_POINT ( 'NONE',  ( 5.000000000000000000, -2.909297654740273256E-16, -7.000000000000000000 ) ) ;
#64757=CARTESIAN_POINT ( 'NONE',  ( 2.241241388159942801E-47, 3.851859888774471706E-31, 7.000000000000000000 ) ) ;
#64772=EDGE_LOOP ( 'NONE', ( #84732, #47102, #82863, #43318 ) ) ;
#64873=DIRECTION ( 'NONE',  ( 0.000000000000000000, 0.000000000000000000, -1.000000000000000000 ) ) ;
#64992=DIRECTION ( 'NONE',  ( 1.000000000000000000, -5.818595309480552676E-17, 0.000000000000000000 ) ) ;
#65078=ORIENTED_EDGE ( 'NONE', *, *, #71522, .T. ) ;
#65105=ORIENTED_EDGE ( 'NONE', *, *, #38299, .F. ) ;
#65111=CARTESIAN_POINT ( 'NONE',  ( 34.56412365047464874, 28.99999999999999645, -7.000000000000000888 ) ) ;
#65128=CARTESIAN_POINT ( 'NONE',  ( 66.76470751278411342, 40.99999999999997868, -9.500000000000000000 ) ) ;
#65166=DIRECTION ( 'NONE',  ( -1.000000000000000000, 0.000000000000000000, 0.000000000000000000 ) ) ;
#65188=ORIENTED_EDGE ( 'NONE', *, *, #89283, .T. ) ;
#65246=DIRECTION ( 'NONE',  ( -1.000000000000000000, 0.000000000000000000, 0.000000000000000000 ) ) ;
#65258=FACE_OUTER_BOUND ( 'NONE', #68662, .T. ) ;
#65283=EDGE_CURVE ( 'NONE', #62023, #92057, #96629, .T. ) ;
#65321=VECTOR ( 'NONE', #39759, 1000.000000000000000 ) ;
#65380=EDGE_CURVE ( 'NONE', #66734, #75199, #42917, .T. ) ;
#65393=EDGE_CURVE ( 'NONE', #18967, #48000, #18942, .T. ) ;
#65430=ORIENTED_EDGE ( 'NONE', *, *, #31881, .T. ) ;
#65461=ORIENTED_EDGE ( 'NONE', *, *, #7847, .F. ) ;
#65473=CIRCLE ( 'NONE', #17616, 0.5000000000000004441 ) ;
#65477=ORIENTED_EDGE ( 'NONE', *, *, #27712, .T. ) ;
#65543=CYLINDRICAL_SURFACE ( 'NONE', #59972, 0.5000000000000002220 ) ;
#65555=VECTOR ( 'NONE', #23501, 1000.000000000000000 ) ;
#65557=CARTESIAN_POINT ( 'NONE',  ( 0.4195498155886434599, -2.441190589077521466E-17, 10.00000000000000000 ) ) ;
#65561=EDGE_LOOP ( 'NONE', ( #35424, #64006, #28096, #33383 ) ) ;
#65600=VERTEX_POINT ( 'NONE', #10939 ) ;
#65605=EDGE_LOOP ( 'NONE', ( #16744, #75699, #97730, #65477 ) ) ;
#65657=TOROIDAL_SURFACE ( 'NONE', #89581, 2.500000000000000888, 0.5000000000000000000 ) ;
#65689=CARTESIAN_POINT ( 'NONE',  ( 24.35999999999999233, 37.99999999999997868, -7.000000000000000888 ) ) ;
#65690=EDGE_CURVE ( 'NONE', #15070, #68783, #74380, .T. ) ;
#65751=EDGE_CURVE ( 'NONE', #28589, #42131, #435, .T. ) ;
#65838=CIRCLE ( 'NONE', #16331, 0.5000000000000004441 ) ;
#65873=LINE ( 'NONE', #88884, #48360 ) ;
#65966=CARTESIAN_POINT ( 'NONE',  ( 32.06412365047463453, 26.99999999999998224, -9.500000000000000000 ) ) ;
#66050=AXIS2_PLACEMENT_3D ( 'NONE', #25729, #58156, #50172 ) ;
#66129=DIRECTION ( 'NONE',  ( 0.000000000000000000, 0.000000000000000000, 1.000000000000000000 ) ) ;
#66134=LINE ( 'NONE', #43637, #56740 ) ;
#66153=EDGE_LOOP ( 'NONE', ( #2884, #43903, #55551, #93515, #3466, #32110, #12809, #63240 ) ) ;
#66170=CARTESIAN_POINT ( 'NONE',  ( 31.00000000000000355, 44.99999999999999289, -7.000000000000000000 ) ) ;
#66175=ORIENTED_EDGE ( 'NONE', *, *, #88613, .T. ) ;
#66203=DIRECTION ( 'NONE',  ( -0.000000000000000000, -0.000000000000000000, -1.000000000000000000 ) ) ;
#66253=DIRECTION ( 'NONE',  ( 8.673617379884027583E-16, 1.000000000000000000, -0.000000000000000000 ) ) ;
#66323=CARTESIAN_POINT ( 'NONE',  ( 69.60148758828985649, 0.4999999999999935052, -9.500000000000000000 ) ) ;
#66339=ORIENTED_EDGE ( 'NONE', *, *, #21522, .F. ) ;
#66368=EDGE_LOOP ( 'NONE', ( #69511, #22350, #65105, #31562, #76608, #7451, #5354, #4133, #59551 ) ) ;
#66395=CARTESIAN_POINT ( 'NONE',  ( -2.614810775378867191, 35.00346125376525919, -9.500000000000000000 ) ) ;
#66420=CARTESIAN_POINT ( 'NONE',  ( 0.4195498155886434599, 0.4999999999999998890, -9.500000000000000000 ) ) ;
#66421=VERTEX_POINT ( 'NONE', #93705 ) ;
#66451=VERTEX_POINT ( 'NONE', #70732 ) ;
#66580=VERTEX_POINT ( 'NONE', #48200 ) ;
#66603=CARTESIAN_POINT ( 'NONE',  ( 38.04706783004212411, 28.99999999999999645, 7.000000000000000000 ) ) ;
#66632=PRODUCT_DEFINITION ( 'UNKNOWN', '', #842, #36482 ) ;
#66649=ORIENTED_EDGE ( 'NONE', *, *, #39878, .F. ) ;
#66714=DIRECTION ( 'NONE',  ( -5.818595309480553908E-17, -1.000000000000000000, -0.000000000000000000 ) ) ;
#66727=FACE_BOUND ( 'NONE', #44353, .T. ) ;
#66734=VERTEX_POINT ( 'NONE', #64659 ) ;
#66865=LINE ( 'NONE', #34881, #27340 ) ;
#66957=VECTOR ( 'NONE', #23641, 1000.000000000000000 ) ;
#67054=DIRECTION ( 'NONE',  ( 0.000000000000000000, 0.000000000000000000, -1.000000000000000000 ) ) ;
#67059=EDGE_CURVE ( 'NONE', #23929, #4006, #65473, .T. ) ;
#67069=VERTEX_POINT ( 'NONE', #67655 ) ;
#67135=VECTOR ( 'NONE', #67384, 1000.000000000000000 ) ;
#67239=DIRECTION ( 'NONE',  ( -1.000000000000000000, 0.000000000000000000, 0.000000000000000000 ) ) ;
#67270=CARTESIAN_POINT ( 'NONE',  ( -0.4957494408796453977, 15.11603861882761812, 9.500000000000000000 ) ) ;
#67287=CARTESIAN_POINT ( 'NONE',  ( 32.06412365047463453, 22.49999999999998934, -10.00000000000000000 ) ) ;
#67305=EDGE_CURVE ( 'NONE', #66734, #49892, #49005, .T. ) ;
#67341=CARTESIAN_POINT ( 'NONE',  ( 0.000000000000000000, 0.000000000000000000, 0.000000000000000000 ) ) ;
#67366=LINE ( 'NONE', #21377, #57668 ) ;
#67369=CARTESIAN_POINT ( 'NONE',  ( 5.000000000000000888, 16.50982297312471303, -7.000000000000000000 ) ) ;
#67384=DIRECTION ( 'NONE',  ( -0.000000000000000000, -0.000000000000000000, 1.000000000000000000 ) ) ;
#67420=ADVANCED_FACE ( 'NONE', ( #54596 ), #18684, .T. ) ;
#67430=CARTESIAN_POINT ( 'NONE',  ( 70.00000000000000000, -4.073016716636387686E-15, -9.500000000000000000 ) ) ;
#67459=EDGE_CURVE ( 'NONE', #77584, #48019, #62095, .T. ) ;
#67540=DIRECTION ( 'NONE',  ( -1.000000000000000000, 5.782411586589362323E-17, -0.000000000000000000 ) ) ;
#67579=ORIENTED_EDGE ( 'NONE', *, *, #32559, .T. ) ;
#67655=CARTESIAN_POINT ( 'NONE',  ( 64.56412365047461321, 29.00000000000000355, -7.000000000000000000 ) ) ;
#67658=FACE_BOUND ( 'NONE', #84952, .T. ) ;
#67706=CIRCLE ( 'NONE', #66050, 2.000000000000001776 ) ;
#67831=DIRECTION ( 'NONE',  ( -5.818595309480553908E-17, -1.000000000000000000, -0.000000000000000000 ) ) ;
#67846=SURFACE_STYLE_USAGE ( .BOTH. , #31300 ) ;
#67910=ORIENTED_EDGE ( 'NONE', *, *, #75674, .T. ) ;
#67911=AXIS2_PLACEMENT_3D ( 'NONE', #46298, #38801, #821 ) ;
#68008=ORIENTED_EDGE ( 'NONE', *, *, #45168, .T. ) ;
#68011=FACE_OUTER_BOUND ( 'NONE', #77927, .T. ) ;
#68078=EDGE_CURVE ( 'NONE', #48000, #41634, #26730, .T. ) ;
#68147=AXIS2_PLACEMENT_3D ( 'NONE', #48784, #41319, #25807 ) ;
#68148=EDGE_CURVE ( 'NONE', #87399, #34693, #1221, .T. ) ;
#68189=EDGE_LOOP ( 'NONE', ( #88664, #61054, #3235 ) ) ;
#68200=CARTESIAN_POINT ( 'NONE',  ( 66.76470751278411342, 44.49999999999998579, 10.00000000000000000 ) ) ;
#68202=LINE ( 'NONE', #7201, #92408 ) ;
#68412=ORIENTED_EDGE ( 'NONE', *, *, #86386, .F. ) ;
#68435=VECTOR ( 'NONE', #84271, 1000.000000000000000 ) ;
#68463=UNCERTAINTY_MEASURE_WITH_UNIT (LENGTH_MEASURE( 1.000000000000000082E-05 ), #92308, 'distance_accuracy_value', 'NONE');
#68464=DIRECTION ( 'NONE',  ( -1.000000000000000000, 0.000000000000000000, 0.000000000000000000 ) ) ;
#68505=CARTESIAN_POINT ( 'NONE',  ( 56.78206182523731371, 44.99999999999999289, 0.000000000000000000 ) ) ;
#68545=VERTEX_POINT ( 'NONE', #50298 ) ;
#68587=LINE ( 'NONE', #14614, #1830 ) ;
#68662=EDGE_LOOP ( 'NONE', ( #84780, #330, #43165, #19145 ) ) ;
#68672=ORIENTED_EDGE ( 'NONE', *, *, #1855, .T. ) ;
#68737=EDGE_LOOP ( 'NONE', ( #30125, #77645, #55148, #6085 ) ) ;
#68750=DIRECTION ( 'NONE',  ( 8.673617379884027583E-16, 1.000000000000000000, 0.000000000000000000 ) ) ;
#68754=AXIS2_PLACEMENT_3D ( 'NONE', #85583, #61583, #25097 ) ;
#68778=CARTESIAN_POINT ( 'NONE',  ( 17.59846011966563850, 33.99402920976537246, 9.945641156544798633 ) ) ;
#68783=VERTEX_POINT ( 'NONE', #44282 ) ;
#68784=EDGE_CURVE ( 'NONE', #11334, #35983, #30890, .T. ) ;
#68791=EDGE_LOOP ( 'NONE', ( #54554, #62626, #19192, #21588 ) ) ;
#68822=FACE_OUTER_BOUND ( 'NONE', #92535, .T. ) ;
#68833=AXIS2_PLACEMENT_3D ( 'NONE', #90969, #76473, #7000 ) ;
#68843=DIRECTION ( 'NONE',  ( -0.000000000000000000, -0.000000000000000000, -1.000000000000000000 ) ) ;
#68847=DIRECTION ( 'NONE',  ( 6.938893903907221278E-15, -1.000000000000000000, 0.000000000000000000 ) ) ;
#68849=DIRECTION ( 'NONE',  ( 1.000000000000000000, -5.818595309480553908E-17, 0.000000000000000000 ) ) ;
#68913=DIRECTION ( 'NONE',  ( -1.000000000000000000, 5.818595309480552676E-17, 0.000000000000000000 ) ) ;
#68943=CARTESIAN_POINT ( 'NONE',  ( 34.56412365047463453, 13.99999999999999645, 10.00000000000000000 ) ) ;
#68961=FACE_OUTER_BOUND ( 'NONE', #85270, .T. ) ;
#68996=CARTESIAN_POINT ( 'NONE',  ( 64.56412365047461321, 11.99999999999999467, 10.00000000000000000 ) ) ;
#69118=DIRECTION ( 'NONE',  ( -1.000000000000000000, 0.000000000000000000, 0.000000000000000000 ) ) ;
#69214=CARTESIAN_POINT ( 'NONE',  ( -27.43587634952537968, 11.50000000000000000, -10.00000000000000000 ) ) ;
#69260=VERTEX_POINT ( 'NONE', #64682 ) ;
#69274=EDGE_CURVE ( 'NONE', #18090, #83143, #50691, .T. ) ;
#69275=ORIENTED_EDGE ( 'NONE', *, *, #22774, .T. ) ;
#69328=CARTESIAN_POINT ( 'NONE',  ( 32.56412365047463453, 26.99999999999998224, 10.00000000000000000 ) ) ;
#69339=FACE_OUTER_BOUND ( 'NONE', #1641, .T. ) ;
#69511=ORIENTED_EDGE ( 'NONE', *, *, #23968, .T. ) ;
#69551=EDGE_CURVE ( 'NONE', #38557, #29252, #71515, .T. ) ;
#69576=LINE ( 'NONE', #76573, #47350 ) ;
#69577=AXIS2_PLACEMENT_3D ( 'NONE', #98260, #743, #31196 ) ;
#69887=ORIENTED_EDGE ( 'NONE', *, *, #43446, .T. ) ;
#69937=DIRECTION ( 'NONE',  ( -1.000000000000000000, 0.000000000000000000, 0.000000000000000000 ) ) ;
#69999=ORIENTED_EDGE ( 'NONE', *, *, #14598, .F. ) ;
#70030=ADVANCED_FACE ( 'NONE', ( #19089, #27069 ), #34071, .F. ) ;
#70056=CIRCLE ( 'NONE', #34923, 19.99999999999999645 ) ;
#70150=CARTESIAN_POINT ( 'NONE',  ( 34.56412365047464874, 29.50000000000000000, 10.00000000000000000 ) ) ;
#70157=ORIENTED_EDGE ( 'NONE', *, *, #14925, .F. ) ;
#70304=AXIS2_PLACEMENT_3D ( 'NONE', #96231, #88213, #27710 ) ;
#70315=DIRECTION ( 'NONE',  ( 0.2211055276381909129, 0.9752498888222635998, -0.000000000000000000 ) ) ;
#70338=CARTESIAN_POINT ( 'NONE',  ( 34.56412365047464874, 11.49999999999999645, 9.500000000000000000 ) ) ;
#70418=DIRECTION ( 'NONE',  ( 1.000000000000000000, 0.000000000000000000, 0.000000000000000000 ) ) ;
#70482=ORIENTED_EDGE ( 'NONE', *, *, #73156, .F. ) ;
#70483=CARTESIAN_POINT ( 'NONE',  ( 0.000000000000000000, 0.000000000000000000, 10.00000000000000000 ) ) ;
#70510=CYLINDRICAL_SURFACE ( 'NONE', #25560, 19.99999999999999645 ) ;
#70564=ADVANCED_FACE ( 'NONE', ( #47496 ), #40006, .T. ) ;
#70582=DIRECTION ( 'NONE',  ( -0.000000000000000000, -0.000000000000000000, -1.000000000000000000 ) ) ;
#70606=DIRECTION ( 'NONE',  ( 0.000000000000000000, 0.000000000000000000, -1.000000000000000000 ) ) ;
#70608=DIRECTION ( 'NONE',  ( -1.000000000000000000, 0.000000000000000000, 0.000000000000000000 ) ) ;
#70684=ORIENTED_EDGE ( 'NONE', *, *, #62760, .T. ) ;
#70732=CARTESIAN_POINT ( 'NONE',  ( 32.56412365047463453, 14.00000000000001066, 9.500000000000000000 ) ) ;
#70772=ORIENTED_EDGE ( 'NONE', *, *, #39660, .T. ) ;
#70829=ORIENTED_EDGE ( 'NONE', *, *, #54653, .T. ) ;
#70949=EDGE_LOOP ( 'NONE', ( #16719, #68008, #35316, #40860 ) ) ;
#70961=DIRECTION ( 'NONE',  ( 0.000000000000000000, 0.000000000000000000, 1.000000000000000000 ) ) ;
#71110=VECTOR ( 'NONE', #66253, 1000.000000000000000 ) ;
#71162=SPHERICAL_SURFACE ( 'NONE', #45071, 0.5000000000000000000 ) ;
#71170=CYLINDRICAL_SURFACE ( 'NONE', #92054, 0.5000000000000004441 ) ;
#71210=ORIENTED_EDGE ( 'NONE', *, *, #38127, .F. ) ;
#71219=DIRECTION ( 'NONE',  ( -0.000000000000000000, -0.000000000000000000, 1.000000000000000000 ) ) ;
#71268=EDGE_CURVE ( 'NONE', #27691, #94289, #73256, .T. ) ;
#71292=CIRCLE ( 'NONE', #20171, 100.0000000000000000 ) ;
#71306=LINE ( 'NONE', #2825, #16339 ) ;
#71310=DIRECTION ( 'NONE',  ( 0.000000000000000000, 0.000000000000000000, 1.000000000000000000 ) ) ;
#71311=CYLINDRICAL_SURFACE ( 'NONE', #68147, 1.999999999999996669 ) ;
#71386=ORIENTED_EDGE ( 'NONE', *, *, #8376, .T. ) ;
#71425=AXIS2_PLACEMENT_3D ( 'NONE', #23080, #102, #59577 ) ;
#71474=CARTESIAN_POINT ( 'NONE',  ( 64.56412365047461321, 28.99999999999999645, 10.00000000000000000 ) ) ;
#71486=ORIENTED_EDGE ( 'NONE', *, *, #49678, .T. ) ;
#71515=CIRCLE ( 'NONE', #23627, 0.5000000000000000000 ) ;
#71522=EDGE_CURVE ( 'NONE', #42904, #40747, #40278, .T. ) ;
#71533=ORIENTED_EDGE ( 'NONE', *, *, #79500, .T. ) ;
#71570=CARTESIAN_POINT ( 'NONE',  ( -2.253458813454140675, 12.77999999999999936, -9.500000000000000000 ) ) ;
#71571=ADVANCED_FACE ( 'NONE', ( #47768 ), #46782, .T. ) ;
#71584=CARTESIAN_POINT ( 'NONE',  ( 38.04706783004212411, 29.00000000000000355, -7.000000000000000000 ) ) ;
#71659=DIRECTION ( 'NONE',  ( -0.000000000000000000, -0.000000000000000000, -1.000000000000000000 ) ) ;
#71707=ORIENTED_EDGE ( 'NONE', *, *, #12686, .T. ) ;
#71756=CARTESIAN_POINT ( 'NONE',  ( 26.00000000000000355, 35.99999999999997158, -7.000000000000000000 ) ) ;
#71778=CARTESIAN_POINT ( 'NONE',  ( 32.26500600480481040, 44.99999999999999289, 0.000000000000000000 ) ) ;
#71855=VECTOR ( 'NONE', #72290, 1000.000000000000000 ) ;
#71861=FACE_OUTER_BOUND ( 'NONE', #29141, .T. ) ;
#71898=EDGE_LOOP ( 'NONE', ( #25726, #15928, #7470, #24843 ) ) ;
#71942=DIRECTION ( 'NONE',  ( 0.000000000000000000, 0.000000000000000000, 1.000000000000000000 ) ) ;
#71981=AXIS2_PLACEMENT_3D ( 'NONE', #63647, #18663, #49151 ) ;
#72034=DIRECTION ( 'NONE',  ( 0.000000000000000000, 1.000000000000000000, 0.000000000000000000 ) ) ;
#72048=VECTOR ( 'NONE', #82510, 1000.000000000000000 ) ;
#72063=ADVANCED_FACE ( 'NONE', ( #22215 ), #22707, .F. ) ;
#72078=FACE_BOUND ( 'NONE', #51699, .T. ) ;
#72079=CARTESIAN_POINT ( 'NONE',  ( 34.56412365047464874, 28.99999999999999645, 10.00000000000000000 ) ) ;
#72095=VECTOR ( 'NONE', #31202, 1000.000000000000000 ) ;
#72183=DIRECTION ( 'NONE',  ( 0.000000000000000000, 0.000000000000000000, -1.000000000000000000 ) ) ;
#72284=ORIENTED_EDGE ( 'NONE', *, *, #4631, .F. ) ;
#72290=DIRECTION ( 'NONE',  ( 0.1736481776669272503, -0.9848077530122086864, 0.000000000000000000 ) ) ;
#72330=VECTOR ( 'NONE', #16099, 1000.000000000000000 ) ;
#72358=AXIS2_PLACEMENT_3D ( 'NONE', #17703, #40689, #1239 ) ;
#72512=EDGE_LOOP ( 'NONE', ( #74453, #1292, #19262 ) ) ;
#72602=EDGE_CURVE ( 'NONE', #4006, #45903, #71292, .T. ) ;
#72661=CARTESIAN_POINT ( 'NONE',  ( -27.43587634952537968, 0.5000000000000038858, 9.500000000000000000 ) ) ;
#72664=ORIENTED_EDGE ( 'NONE', *, *, #49558, .F. ) ;
#72774=CARTESIAN_POINT ( 'NONE',  ( 67.06412365047464164, 14.00000000000000888, 10.00000000000000000 ) ) ;
#72808=VECTOR ( 'NONE', #89841, 1000.000000000000000 ) ;
#72850=AXIS2_PLACEMENT_3D ( 'NONE', #62571, #62077, #40585 ) ;
#72880=FACE_OUTER_BOUND ( 'NONE', #63978, .T. ) ;
#72903=CARTESIAN_POINT ( 'NONE',  ( 34.56412365047464874, 11.49999999999999645, -9.500000000000000000 ) ) ;
#73146=ORIENTED_EDGE ( 'NONE', *, *, #4170, .F. ) ;
#73156=EDGE_CURVE ( 'NONE', #22113, #295, #71306, .T. ) ;
#73225=DIRECTION ( 'NONE',  ( 1.000000000000000000, 0.000000000000000000, 0.000000000000000000 ) ) ;
#73238=DIRECTION ( 'NONE',  ( -0.000000000000000000, -0.000000000000000000, -1.000000000000000000 ) ) ;
#73256=CIRCLE ( 'NONE', #1429, 1.500000000000001332 ) ;
#73349=VECTOR ( 'NONE', #24501, 1000.000000000000000 ) ;
#73354=ORIENTED_EDGE ( 'NONE', *, *, #92279, .F. ) ;
#73418=AXIS2_PLACEMENT_3D ( 'NONE', #94853, #26354, #75302 ) ;
#73480=EDGE_LOOP ( 'NONE', ( #46551, #58692, #96792, #47130 ) ) ;
#73505=VECTOR ( 'NONE', #22130, 1000.000000000000000 ) ;
#73553=EDGE_CURVE ( 'NONE', #83062, #10816, #85002, .T. ) ;
#73559=CIRCLE ( 'NONE', #12687, 6.999999999999995559 ) ;
#73580=ADVANCED_FACE ( 'NONE', ( #2744 ), #19190, .T. ) ;
#73619=CARTESIAN_POINT ( 'NONE',  ( 64.56412365047461321, 11.49999999999999467, 9.500000000000000000 ) ) ;
#73688=ORIENTED_EDGE ( 'NONE', *, *, #46181, .T. ) ;
#73713=DIRECTION ( 'NONE',  ( -1.000000000000000000, 0.000000000000000000, 0.000000000000000000 ) ) ;
#73747=DIRECTION ( 'NONE',  ( -5.818595309480553908E-17, -1.000000000000000000, 0.000000000000000000 ) ) ;
#73764=DIRECTION ( 'NONE',  ( -1.000000000000000000, 5.782411586589362323E-17, 0.000000000000000000 ) ) ;
#73821=ADVANCED_FACE ( 'NONE', ( #67658, #20669, #37164 ), #83140, .F. ) ;
#73833=CARTESIAN_POINT ( 'NONE',  ( -0.2838433074297238012, 13.12729635533385597, 9.500000000000000000 ) ) ;
#73900=VECTOR ( 'NONE', #89887, 1000.000000000000000 ) ;
#74171=EDGE_CURVE ( 'NONE', #25854, #13186, #62498, .T. ) ;
#74318=DIRECTION ( 'NONE',  ( -0.000000000000000000, -0.000000000000000000, -1.000000000000000000 ) ) ;
#74375=DIRECTION ( 'NONE',  ( -1.000000000000000000, 0.000000000000000000, 0.000000000000000000 ) ) ;
#74380=LINE ( 'NONE', #5907, #73900 ) ;
#74403=ORIENTED_EDGE ( 'NONE', *, *, #58413, .T. ) ;
#74445=VECTOR ( 'NONE', #24339, 1000.000000000000000 ) ;
#74453=ORIENTED_EDGE ( 'NONE', *, *, #94367, .F. ) ;
#74469=PLANE ( 'NONE',  #44612 ) ;
#74507=PLANE ( 'NONE',  #87964 ) ;
#74566=ORIENTED_EDGE ( 'NONE', *, *, #7017, .T. ) ;
#74581=ORIENTED_EDGE ( 'NONE', *, *, #94315, .F. ) ;
#74614=VECTOR ( 'NONE', #1777, 1000.000000000000000 ) ;
#74718=FACE_BOUND ( 'NONE', #32709, .T. ) ;
#74732=DIRECTION ( 'NONE',  ( -0.000000000000000000, -0.000000000000000000, -1.000000000000000000 ) ) ;
#74740=DIRECTION ( 'NONE',  ( 1.000000000000000000, 0.000000000000000000, 0.000000000000000000 ) ) ;
#74781=CARTESIAN_POINT ( 'NONE',  ( 0.4195498155886338565, 0.5000000000000023315, 10.00000000000000000 ) ) ;
#74886=CARTESIAN_POINT ( 'NONE',  ( 66.76470751278411342, 44.49999999999998579, -9.500000000000000000 ) ) ;
#74905=ORIENTED_EDGE ( 'NONE', *, *, #41909, .T. ) ;
#74978=CARTESIAN_POINT ( 'NONE',  ( 70.19910379943081580, 41.67447916666664298, -10.00000000000000000 ) ) ;
#75015=ORIENTED_EDGE ( 'NONE', *, *, #67305, .F. ) ;
#75029=ORIENTED_EDGE ( 'NONE', *, *, #14061, .F. ) ;
#75088=CARTESIAN_POINT ( 'NONE',  ( 17.35999999999999943, 37.99999999999997868, 10.00000000000000000 ) ) ;
#75163=VECTOR ( 'NONE', #55055, 1000.000000000000000 ) ;
#75199=VERTEX_POINT ( 'NONE', #92543 ) ;
#75244=DIRECTION ( 'NONE',  ( 0.000000000000000000, 1.000000000000000000, 0.000000000000000000 ) ) ;
#75302=DIRECTION ( 'NONE',  ( -1.000000000000000000, 0.000000000000000000, 0.000000000000000000 ) ) ;
#75398=CARTESIAN_POINT ( 'NONE',  ( 24.35999999999999233, 37.99999999999997868, 10.00000000000000000 ) ) ;
#75400=TOROIDAL_SURFACE ( 'NONE', #11521, 1.499999999999996669, 0.5000000000000000000 ) ;
#75440=AXIS2_PLACEMENT_3D ( 'NONE', #44019, #97553, #59524 ) ;
#75447=DIRECTION ( 'NONE',  ( -1.000000000000000000, 0.000000000000000000, 0.000000000000000000 ) ) ;
#75457=DIRECTION ( 'NONE',  ( -0.000000000000000000, -0.000000000000000000, 1.000000000000000000 ) ) ;
#75481=ORIENTED_EDGE ( 'NONE', *, *, #72602, .T. ) ;
#75536=ADVANCED_FACE ( 'NONE', ( #17459 ), #62935, .T. ) ;
#75583=CARTESIAN_POINT ( 'NONE',  ( 27.50000000000000355, 35.99999999999997158, -10.00000000000000000 ) ) ;
#75595=ORIENTED_EDGE ( 'NONE', *, *, #54855, .F. ) ;
#75663=ORIENTED_EDGE ( 'NONE', *, *, #15488, .T. ) ;
#75674=EDGE_CURVE ( 'NONE', #66451, #6038, #65838, .T. ) ;
#75699=ORIENTED_EDGE ( 'NONE', *, *, #28828, .T. ) ;
#75738=CARTESIAN_POINT ( 'NONE',  ( 69.60148758828984228, 0.4999999999999982792, 9.500000000000000000 ) ) ;
#75768=ADVANCED_FACE ( 'NONE', ( #4907 ), #44852, .T. ) ;
#75791=ORIENTED_EDGE ( 'NONE', *, *, #11802, .F. ) ;
#75802=VERTEX_POINT ( 'NONE', #67369 ) ;
#75810=FACE_OUTER_BOUND ( 'NONE', #71898, .T. ) ;
#75833=TOROIDAL_SURFACE ( 'NONE', #93462, 2.500000000000001776, 0.5000000000000000000 ) ;
#75845=DIRECTION ( 'NONE',  ( -1.000000000000000000, 0.000000000000000000, 0.000000000000000000 ) ) ;
#75853=CARTESIAN_POINT ( 'NONE',  ( 24.35999999999999233, 44.99999999999997868, 10.00000000000000000 ) ) ;
#75924=AXIS2_PLACEMENT_3D ( 'NONE', #39726, #31706, #9709 ) ;
#75994=TOROIDAL_SURFACE ( 'NONE', #47221, 2.500000000000001776, 0.5000000000000000000 ) ;
#76087=ADVANCED_FACE ( 'NONE', ( #16345 ), #54813, .F. ) ;
#76107=DIRECTION ( 'NONE',  ( -5.818595309480553908E-17, -1.000000000000000000, 0.000000000000000000 ) ) ;
#76113=TOROIDAL_SURFACE ( 'NONE', #56904, 20.49999999999999645, 0.5000000000000000000 ) ;
#76172=ORIENTED_EDGE ( 'NONE', *, *, #1722, .F. ) ;
#76197=DIRECTION ( 'NONE',  ( -0.000000000000000000, -0.000000000000000000, -1.000000000000000000 ) ) ;
#76209=AXIS2_PLACEMENT_3D ( 'NONE', #52521, #43057, #98052 ) ;
#76217=CARTESIAN_POINT ( 'NONE',  ( 64.56412365047461321, 28.99999999999999645, -9.500000000000000000 ) ) ;
#76260=ORIENTED_EDGE ( 'NONE', *, *, #80594, .F. ) ;
#76301=CARTESIAN_POINT ( 'NONE',  ( 32.56412365047463453, 14.00000000000001066, 9.500000000000000000 ) ) ;
#76323=EDGE_CURVE ( 'NONE', #81201, #93263, #40328, .T. ) ;
#76337=CARTESIAN_POINT ( 'NONE',  ( 24.35999999999999233, 37.99999999999997868, 10.00000000000000000 ) ) ;
#76352=DIRECTION ( 'NONE',  ( 0.000000000000000000, 0.000000000000000000, 1.000000000000000000 ) ) ;
#76470=CARTESIAN_POINT ( 'NONE',  ( 34.56412365047464874, 28.99999999999999645, 10.00000000000000000 ) ) ;
#76473=DIRECTION ( 'NONE',  ( 0.000000000000000000, 0.000000000000000000, -1.000000000000000000 ) ) ;
#76479=LINE ( 'NONE', #7993, #65555 ) ;
#76573=CARTESIAN_POINT ( 'NONE',  ( 64.56412365047461321, 44.99999999999998579, -7.000000000000000000 ) ) ;
#76608=ORIENTED_EDGE ( 'NONE', *, *, #45168, .F. ) ;
#76684=CARTESIAN_POINT ( 'NONE',  ( 0.4195498155886434599, -2.441190589077521466E-17, 9.500000000000000000 ) ) ;
#76711=LINE ( 'NONE', #60232, #72095 ) ;
#76733=AXIS2_PLACEMENT_3D ( 'NONE', #10079, #61097, #91607 ) ;
#76744=DIRECTION ( 'NONE',  ( -1.000000000000000000, 0.000000000000000000, 0.000000000000000000 ) ) ;
#76792=CARTESIAN_POINT ( 'NONE',  ( 66.76470751278411342, 44.99999999999998579, 10.00000000000000000 ) ) ;
#76900=CIRCLE ( 'NONE', #46568, 19.99999999999999645 ) ;
#76982=PLANE ( 'NONE',  #81550 ) ;
#76998=CARTESIAN_POINT ( 'NONE',  ( 0.4195498155886434599, -2.441190589077521466E-17, -9.500000000000000000 ) ) ;
#77048=VERTEX_POINT ( 'NONE', #95361 ) ;
#77059=ORIENTED_EDGE ( 'NONE', *, *, #27965, .F. ) ;
#77061=VECTOR ( 'NONE', #4296, 1000.000000000000000 ) ;
#77084=LINE ( 'NONE', #47577, #72330 ) ;
#77109=DIRECTION ( 'NONE',  ( -0.000000000000000000, -0.000000000000000000, 1.000000000000000000 ) ) ;
#77157=EDGE_LOOP ( 'NONE', ( #90996, #7426, #70157, #779 ) ) ;
#77165=CARTESIAN_POINT ( 'NONE',  ( 64.56412365047462742, 13.99999999999999467, -9.500000000000000000 ) ) ;
#77168=DIRECTION ( 'NONE',  ( 0.1736481776669272503, -0.9848077530122086864, 0.000000000000000000 ) ) ;
#77253=ORIENTED_EDGE ( 'NONE', *, *, #88394, .F. ) ;
#77308=DIRECTION ( 'NONE',  ( -1.000000000000000000, 8.673617379884036705E-17, 0.000000000000000000 ) ) ;
#77310=SPHERICAL_SURFACE ( 'NONE', #63493, 0.5000000000000000000 ) ;
#77397=DIRECTION ( 'NONE',  ( -8.673617379884027583E-16, -1.000000000000000000, 0.000000000000000000 ) ) ;
#77413=DIRECTION ( 'NONE',  ( -0.000000000000000000, -0.000000000000000000, -1.000000000000000000 ) ) ;
#77440=DIRECTION ( 'NONE',  ( 0.000000000000000000, -0.000000000000000000, -1.000000000000000000 ) ) ;
#77561=CARTESIAN_POINT ( 'NONE',  ( 32.56412365047463453, 14.00000000000001066, 10.00000000000000000 ) ) ;
#77577=CARTESIAN_POINT ( 'NONE',  ( 26.00000000000000355, 35.99999999999997158, 10.00000000000000000 ) ) ;
#77584=VERTEX_POINT ( 'NONE', #94256 ) ;
#77596=AXIS2_PLACEMENT_3D ( 'NONE', #75398, #53387, #36425 ) ;
#77617=CARTESIAN_POINT ( 'NONE',  ( -0.2838433074297238012, 13.12729635533385597, -9.500000000000000000 ) ) ;
#77645=ORIENTED_EDGE ( 'NONE', *, *, #50461, .F. ) ;
#77671=ADVANCED_FACE ( 'NONE', ( #18773 ), #56278, .T. ) ;
#77710=CARTESIAN_POINT ( 'NONE',  ( 32.56412365047463453, 26.99999999999998224, 9.500000000000000000 ) ) ;
#77793=ADVANCED_FACE ( 'NONE', ( #87737 ), #57239, .F. ) ;
#77830=CYLINDRICAL_SURFACE ( 'NONE', #81549, 2.000000000000001776 ) ;
#77894=EDGE_CURVE ( 'NONE', #26787, #18967, #59640, .T. ) ;
#77927=EDGE_LOOP ( 'NONE', ( #7793, #91633, #1530, #4611 ) ) ;
#77958=ORIENTED_EDGE ( 'NONE', *, *, #13039, .F. ) ;
#77981=VERTEX_POINT ( 'NONE', #29695 ) ;
#78001=FACE_OUTER_BOUND ( 'NONE', #70949, .T. ) ;
#78016=EDGE_CURVE ( 'NONE', #45903, #42131, #52826, .T. ) ;
#78249=VERTEX_POINT ( 'NONE', #76684 ) ;
#78275=CARTESIAN_POINT ( 'NONE',  ( 34.56412365047464874, 11.99999999999999645, 10.00000000000000000 ) ) ;
#78296=TOROIDAL_SURFACE ( 'NONE', #47963, 6.499999999999995559, 0.5000000000000000000 ) ;
#78301=FACE_OUTER_BOUND ( 'NONE', #61042, .T. ) ;
#78346=CIRCLE ( 'NONE', #79908, 1.500000000000001332 ) ;
#78370=ORIENTED_EDGE ( 'NONE', *, *, #97546, .F. ) ;
#78372=CARTESIAN_POINT ( 'NONE',  ( 32.06412365047463453, 26.99999999999997868, 10.00000000000000000 ) ) ;
#78378=AXIS2_PLACEMENT_3D ( 'NONE', #75853, #98885, #5882 ) ;
#78424=CARTESIAN_POINT ( 'NONE',  ( 17.59846011966563850, 33.99402920976536535, -9.945641156544795081 ) ) ;
#78441=FACE_OUTER_BOUND ( 'NONE', #90537, .T. ) ;
#78501=CARTESIAN_POINT ( 'NONE',  ( -1.761054936948033278, 12.86682408883346440, 10.00000000000000000 ) ) ;
#78526=VECTOR ( 'NONE', #49398, 1000.000000000000000 ) ;
#78570=CYLINDRICAL_SURFACE ( 'NONE', #76733, 0.5000000000000004441 ) ;
#78607=LINE ( 'NONE', #72079, #59423 ) ;
#78618=ORIENTED_EDGE ( 'NONE', *, *, #86122, .F. ) ;
#78639=ORIENTED_EDGE ( 'NONE', *, *, #56268, .F. ) ;
#78647=CARTESIAN_POINT ( 'NONE',  ( 32.06412365047463453, 14.00000000000001421, -10.00000000000000000 ) ) ;
#78662=ORIENTED_EDGE ( 'NONE', *, *, #81204, .T. ) ;
#78689=VECTOR ( 'NONE', #87911, 1000.000000000000000 ) ;
#78718=ORIENTED_EDGE ( 'NONE', *, *, #39326, .F. ) ;
#78771=ADVANCED_FACE ( 'NONE', ( #11630 ), #95118, .T. ) ;
#78773=DIRECTION ( 'NONE',  ( -0.000000000000000000, -0.000000000000000000, -1.000000000000000000 ) ) ;
#78782=EDGE_CURVE ( 'NONE', #66580, #10785, #51196, .T. ) ;
#78868=VERTEX_POINT ( 'NONE', #30071 ) ;
#78937=DIRECTION ( 'NONE',  ( -1.000000000000000000, 0.000000000000000000, 0.000000000000000000 ) ) ;
#79008=ADVANCED_FACE ( 'NONE', ( #83587 ), #22103, .F. ) ;
#79013=CARTESIAN_POINT ( 'NONE',  ( -0.2838433074297238012, 13.12729635533385597, 9.500000000000000000 ) ) ;
#79044=EDGE_CURVE ( 'NONE', #46560, #83062, #68587, .T. ) ;
#79090=DIRECTION ( 'NONE',  ( -0.000000000000000000, -0.000000000000000000, -1.000000000000000000 ) ) ;
#79129=ORIENTED_EDGE ( 'NONE', *, *, #84120, .F. ) ;
#79141=DIRECTION ( 'NONE',  ( 0.000000000000000000, 1.000000000000000000, 0.000000000000000000 ) ) ;
#79226=CIRCLE ( 'NONE', #61647, 1.500000000000001332 ) ;
#79251=EDGE_CURVE ( 'NONE', #25266, #62023, #50519, .T. ) ;
#79303=CIRCLE ( 'NONE', #58594, 2.000000000000001776 ) ;
#79387=DIRECTION ( 'NONE',  ( 0.000000000000000000, 0.000000000000000000, 1.000000000000000000 ) ) ;
#79391=VECTOR ( 'NONE', #21779, 1000.000000000000000 ) ;
#79410=CARTESIAN_POINT ( 'NONE',  ( 56.78206182523731371, 28.99999999999999645, 0.000000000000000000 ) ) ;
#79500=EDGE_CURVE ( 'NONE', #50694, #11231, #43257, .T. ) ;
#79515=ORIENTED_EDGE ( 'NONE', *, *, #57225, .F. ) ;
#79602=ORIENTED_EDGE ( 'NONE', *, *, #21940, .T. ) ;
#79640=CARTESIAN_POINT ( 'NONE',  ( 70.00000000000000000, 0.4999999999999958922, -9.500000000000000000 ) ) ;
#79667=DIRECTION ( 'NONE',  ( -0.000000000000000000, -0.000000000000000000, -1.000000000000000000 ) ) ;
#79735=VECTOR ( 'NONE', #94079, 1000.000000000000000 ) ;
#79789=DIRECTION ( 'NONE',  ( 1.000000000000000000, 0.000000000000000000, 0.000000000000000000 ) ) ;
#79860=ORIENTED_EDGE ( 'NONE', *, *, #79251, .F. ) ;
#79908=AXIS2_PLACEMENT_3D ( 'NONE', #29373, #90864, #74375 ) ;
#79957=DIRECTION ( 'NONE',  ( 1.000000000000000000, -5.818595309480553908E-17, 0.000000000000000000 ) ) ;
#79967=ORIENTED_EDGE ( 'NONE', *, *, #22911, .T. ) ;
#80050=DIRECTION ( 'NONE',  ( 0.000000000000000000, -1.000000000000000000, 0.000000000000000000 ) ) ;
#80068=ORIENTED_EDGE ( 'NONE', *, *, #5431, .T. ) ;
#80085=CARTESIAN_POINT ( 'NONE',  ( 66.56412365047464164, 14.00000000000000888, -9.500000000000000000 ) ) ;
#80086=ORIENTED_EDGE ( 'NONE', *, *, #42026, .F. ) ;
#80132=EDGE_CURVE ( 'NONE', #27691, #47516, #25453, .T. ) ;
#80228=CIRCLE ( 'NONE', #43466, 0.5000000000000004441 ) ;
#80338=VECTOR ( 'NONE', #82348, 1000.000000000000000 ) ;
#80343=ORIENTED_EDGE ( 'NONE', *, *, #8280, .T. ) ;
#80390=LINE ( 'NONE', #27377, #62153 ) ;
#80483=AXIS2_PLACEMENT_3D ( 'NONE', #21752, #98757, #37250 ) ;
#80519=DIRECTION ( 'NONE',  ( 1.084202172485504681E-16, 1.000000000000000000, 0.000000000000000000 ) ) ;
#80593=CIRCLE ( 'NONE', #47098, 6.999999999999995559 ) ;
#80594=EDGE_CURVE ( 'NONE', #35183, #20515, #11499, .T. ) ;
#80601=ORIENTED_EDGE ( 'NONE', *, *, #62641, .F. ) ;
#80678=CARTESIAN_POINT ( 'NONE',  ( 0.4195498155886434599, 0.4999999999999998890, 10.00000000000000000 ) ) ;
#80792=CARTESIAN_POINT ( 'NONE',  ( 34.56412365047464874, 28.99999999999999645, 9.500000000000000000 ) ) ;
#80799=CIRCLE ( 'NONE', #52101, 1.500000000000001332 ) ;
#80814=EDGE_LOOP ( 'NONE', ( #13000, #10249, #65430, #33809 ) ) ;
#81054=ORIENTED_EDGE ( 'NONE', *, *, #76323, .T. ) ;
#81127=CARTESIAN_POINT ( 'NONE',  ( 32.06412365047463453, 14.00000000000001066, 10.00000000000000000 ) ) ;
#81159=DIRECTION ( 'NONE',  ( 1.000000000000000000, -5.818595309480552676E-17, 0.000000000000000000 ) ) ;
#81201=VERTEX_POINT ( 'NONE', #51563 ) ;
#81204=EDGE_CURVE ( 'NONE', #78249, #29252, #98070, .T. ) ;
#81212=FACE_OUTER_BOUND ( 'NONE', #32809, .T. ) ;
#81229=DIRECTION ( 'NONE',  ( 1.000000000000000000, -5.818595309480553908E-17, 0.000000000000000000 ) ) ;
#81230=DIRECTION ( 'NONE',  ( -0.000000000000000000, -0.000000000000000000, 1.000000000000000000 ) ) ;
#81278=DIRECTION ( 'NONE',  ( 1.000000000000000000, -5.818595309480553908E-17, 0.000000000000000000 ) ) ;
#81304=VECTOR ( 'NONE', #83463, 1000.000000000000000 ) ;
#81357=CARTESIAN_POINT ( 'NONE',  ( 64.56412365047461321, 11.99999999999999467, 10.00000000000000000 ) ) ;
#81435=DIRECTION ( 'NONE',  ( 1.000000000000000000, 0.000000000000000000, 0.000000000000000000 ) ) ;
#81457=ORIENTED_EDGE ( 'NONE', *, *, #8903, .F. ) ;
#81504=AXIS2_PLACEMENT_3D ( 'NONE', #31578, #70582, #17097 ) ;
#81521=DIRECTION ( 'NONE',  ( -1.000000000000000000, -1.636349903325072848E-16, 0.000000000000000000 ) ) ;
#81523=ORIENTED_EDGE ( 'NONE', *, *, #10767, .T. ) ;
#81549=AXIS2_PLACEMENT_3D ( 'NONE', #15877, #61844, #92350 ) ;
#81550=AXIS2_PLACEMENT_3D ( 'NONE', #84001, #41, #98544 ) ;
#81603=CARTESIAN_POINT ( 'NONE',  ( 34.56412365047464874, 11.99999999999999645, 10.00000000000000000 ) ) ;
#81646=CYLINDRICAL_SURFACE ( 'NONE', #87275, 0.5000000000000000000 ) ;
#81648=CARTESIAN_POINT ( 'NONE',  ( 70.00000000000000000, -4.073016716636387686E-15, 10.00000000000000000 ) ) ;
#81710=CARTESIAN_POINT ( 'NONE',  ( 64.56412365047461321, 44.99999999999998579, 0.000000000000000000 ) ) ;
#81721=EDGE_CURVE ( 'NONE', #62689, #6556, #97831, .T. ) ;
#81757=FACE_OUTER_BOUND ( 'NONE', #20531, .T. ) ;
#81897=AXIS2_PLACEMENT_3D ( 'NONE', #45197, #21219, #37226 ) ;
#81956=CARTESIAN_POINT ( 'NONE',  ( 64.56412365047461321, 44.99999999999998579, 0.000000000000000000 ) ) ;
#82054=VERTEX_POINT ( 'NONE', #45419 ) ;
#82176=( GEOMETRIC_REPRESENTATION_CONTEXT ( 3 ) GLOBAL_UNCERTAINTY_ASSIGNED_CONTEXT ( ( #68463 ) ) GLOBAL_UNIT_ASSIGNED_CONTEXT ( ( #92308, #38827, #44821 ) ) REPRESENTATION_CONTEXT ( 'NONE', 'WORKASPACE' ) );
#82204=EDGE_CURVE ( 'NONE', #30184, #44141, #80228, .T. ) ;
#82319=EDGE_CURVE ( 'NONE', #63645, #78249, #64225, .T. ) ;
#82348=DIRECTION ( 'NONE',  ( 0.000000000000000000, 0.000000000000000000, 1.000000000000000000 ) ) ;
#82406=FACE_OUTER_BOUND ( 'NONE', #77157, .T. ) ;
#82437=DIRECTION ( 'NONE',  ( 0.000000000000000000, 0.000000000000000000, 1.000000000000000000 ) ) ;
#82465=UNCERTAINTY_MEASURE_WITH_UNIT (LENGTH_MEASURE( 1.000000000000000082E-05 ), #45837, 'distance_accuracy_value', 'NONE');
#82507=EDGE_CURVE ( 'NONE', #4006, #55254, #33889, .T. ) ;
#82510=DIRECTION ( 'NONE',  ( -0.000000000000000000, -0.000000000000000000, -1.000000000000000000 ) ) ;
#82530=CARTESIAN_POINT ( 'NONE',  ( 34.56412365047464874, 11.49999999999999645, 10.00000000000000000 ) ) ;
#82579=EDGE_LOOP ( 'NONE', ( #61011, #78662, #48444, #64203 ) ) ;
#82665=EDGE_LOOP ( 'NONE', ( #20319, #40628, #43316, #33596 ) ) ;
#82694=VECTOR ( 'NONE', #26699, 1000.000000000000000 ) ;
#82715=CARTESIAN_POINT ( 'NONE',  ( 66.56412365047464164, 14.00000000000000888, 10.00000000000000000 ) ) ;
#82746=DIRECTION ( 'NONE',  ( -1.000000000000000000, 5.818595309480552676E-17, -0.000000000000000000 ) ) ;
#82753=CARTESIAN_POINT ( 'NONE',  ( 17.85999999999999943, 37.99999999999997868, -9.500000000000000000 ) ) ;
#82769=ORIENTED_EDGE ( 'NONE', *, *, #4764, .F. ) ;
#82796=ORIENTED_EDGE ( 'NONE', *, *, #18867, .F. ) ;
#82842=CARTESIAN_POINT ( 'NONE',  ( 64.56412365047461321, 11.99999999999999467, 6.999999999999999112 ) ) ;
#82846=CARTESIAN_POINT ( 'NONE',  ( -0.2838433074297238012, 13.12729635533385597, 9.500000000000000000 ) ) ;
#82863=ORIENTED_EDGE ( 'NONE', *, *, #348, .F. ) ;
#82911=ORIENTED_EDGE ( 'NONE', *, *, #62975, .F. ) ;
#82954=CARTESIAN_POINT ( 'NONE',  ( 5.000000000000000000, -2.909297654740273256E-16, 0.000000000000000000 ) ) ;
#83025=CIRCLE ( 'NONE', #30263, 1.999999999999996669 ) ;
#83062=VERTEX_POINT ( 'NONE', #3261 ) ;
#83086=DIRECTION ( 'NONE',  ( 8.673617379884027583E-16, 1.000000000000000000, 0.000000000000000000 ) ) ;
#83140=PLANE ( 'NONE',  #88053 ) ;
#83143=VERTEX_POINT ( 'NONE', #10763 ) ;
#83162=ORIENTED_EDGE ( 'NONE', *, *, #31652, .T. ) ;
#83163=DIRECTION ( 'NONE',  ( 0.000000000000000000, 0.000000000000000000, 1.000000000000000000 ) ) ;
#83192=DIRECTION ( 'NONE',  ( -1.000000000000000000, 0.000000000000000000, 0.000000000000000000 ) ) ;
#83226=CARTESIAN_POINT ( 'NONE',  ( 24.35999999999999233, 37.99999999999997868, -9.500000000000000000 ) ) ;
#83293=ORIENTED_EDGE ( 'NONE', *, *, #31051, .F. ) ;
#83297=ORIENTED_EDGE ( 'NONE', *, *, #35159, .F. ) ;
#83350=FACE_OUTER_BOUND ( 'NONE', #14198, .T. ) ;
#83352=DIRECTION ( 'NONE',  ( 0.000000000000000000, 1.000000000000000000, 0.000000000000000000 ) ) ;
#83357=DIRECTION ( 'NONE',  ( 1.000000000000000000, -5.818595309480553908E-17, 0.000000000000000000 ) ) ;
#83361=CARTESIAN_POINT ( 'NONE',  ( 26.00000000000000355, 35.99999999999997158, -10.00000000000000000 ) ) ;
#83391=CARTESIAN_POINT ( 'NONE',  ( 34.56412365047463453, 13.99999999999999645, -9.500000000000000000 ) ) ;
#83408=ORIENTED_EDGE ( 'NONE', *, *, #97546, .T. ) ;
#83416=VECTOR ( 'NONE', #52581, 1000.000000000000000 ) ;
#83445=CYLINDRICAL_SURFACE ( 'NONE', #21287, 0.5000000000000004441 ) ;
#83447=LINE ( 'NONE', #82954, #96225 ) ;
#83452=AXIS2_PLACEMENT_3D ( 'NONE', #66323, #29311, #28818 ) ;
#83463=DIRECTION ( 'NONE',  ( 1.000000000000000000, -0.000000000000000000, -0.000000000000000000 ) ) ;
#83481=DIRECTION ( 'NONE',  ( -0.000000000000000000, -0.000000000000000000, -1.000000000000000000 ) ) ;
#83587=FACE_OUTER_BOUND ( 'NONE', #34494, .T. ) ;
#83660=DIRECTION ( 'NONE',  ( -1.000000000000000000, 0.000000000000000000, 0.000000000000000000 ) ) ;
#83662=ORIENTED_EDGE ( 'NONE', *, *, #63448, .T. ) ;
#83677=ORIENTED_EDGE ( 'NONE', *, *, #58135, .T. ) ;
#83834=DIRECTION ( 'NONE',  ( -0.000000000000000000, 0.000000000000000000, -1.000000000000000000 ) ) ;
#83849=CIRCLE ( 'NONE', #35949, 0.5000000000000000000 ) ;
#83892=ORIENTED_EDGE ( 'NONE', *, *, #1615, .T. ) ;
#83938=DIRECTION ( 'NONE',  ( -0.000000000000000000, -0.000000000000000000, -1.000000000000000000 ) ) ;
#84001=CARTESIAN_POINT ( 'NONE',  ( 64.56412365047461321, 44.99999999999998579, 0.000000000000000000 ) ) ;
#84033=CARTESIAN_POINT ( 'NONE',  ( 66.76470751278411342, 40.99999999999997868, 10.00000000000000000 ) ) ;
#84047=AXIS2_PLACEMENT_3D ( 'NONE', #66420, #11948, #42452 ) ;
#84120=EDGE_CURVE ( 'NONE', #68783, #89049, #93142, .T. ) ;
#84124=CARTESIAN_POINT ( 'NONE',  ( -0.2838433074297238012, 13.12729635533385597, -10.00000000000000000 ) ) ;
#84136=CARTESIAN_POINT ( 'NONE',  ( 24.35999999999999233, 44.49999999999997158, 9.500000000000000000 ) ) ;
#84180=VERTEX_POINT ( 'NONE', #43460 ) ;
#84271=DIRECTION ( 'NONE',  ( -8.673617379884027583E-16, -1.000000000000000000, 0.000000000000000000 ) ) ;
#84294=VECTOR ( 'NONE', #98257, 1000.000000000000000 ) ;
#84328=ADVANCED_FACE ( 'NONE', ( #60928 ), #83445, .T. ) ;
#84334=SHAPE_REPRESENTATION_RELATIONSHIP ( 'NONE' , 'NONE' ,  #53719, #30996 ) ;
#84359=DIRECTION ( 'NONE',  ( 1.000000000000000000, 0.000000000000000000, 0.000000000000000000 ) ) ;
#84432=TOROIDAL_SURFACE ( 'NONE', #41344, 1.499999999999996669, 0.5000000000000000000 ) ;
#84457=PLANE ( 'NONE',  #14979 ) ;
#84501=PLANE ( 'NONE',  #64405 ) ;
#84513=VECTOR ( 'NONE', #86257, 1000.000000000000000 ) ;
#84602=DIRECTION ( 'NONE',  ( 5.818595309480553908E-17, 1.000000000000000000, -0.000000000000000000 ) ) ;
#84700=AXIS2_PLACEMENT_3D ( 'NONE', #34903, #27405, #26916 ) ;
#84732=ORIENTED_EDGE ( 'NONE', *, *, #26876, .T. ) ;
#84780=ORIENTED_EDGE ( 'NONE', *, *, #45124, .T. ) ;
#84805=CIRCLE ( 'NONE', #49668, 2.000000000000001776 ) ;
#84952=EDGE_LOOP ( 'NONE', ( #48227, #72664, #59520, #341 ) ) ;
#84973=AXIS2_PLACEMENT_3D ( 'NONE', #92383, #68913, #23422 ) ;
#85002=CIRCLE ( 'NONE', #14790, 2.000000000000001776 ) ;
#85166=ORIENTED_EDGE ( 'NONE', *, *, #28828, .F. ) ;
#85266=VERTEX_POINT ( 'NONE', #60326 ) ;
#85270=EDGE_LOOP ( 'NONE', ( #13182, #79602, #81457, #17759 ) ) ;
#85281=ORIENTED_EDGE ( 'NONE', *, *, #18867, .T. ) ;
#85303=ADVANCED_FACE ( 'NONE', ( #32771 ), #75833, .T. ) ;
#85320=DIRECTION ( 'NONE',  ( 0.000000000000000000, 0.000000000000000000, -1.000000000000000000 ) ) ;
#85403=ORIENTED_EDGE ( 'NONE', *, *, #24550, .T. ) ;
#85583=CARTESIAN_POINT ( 'NONE',  ( 0.4924038765061043432, 0.08682408883346362516, -9.500000000000000000 ) ) ;
#85661=LINE ( 'NONE', #55660, #61854 ) ;
#85741=CARTESIAN_POINT ( 'NONE',  ( 24.35999999999999233, 37.99999999999997868, 9.500000000000000000 ) ) ;
#85772=LINE ( 'NONE', #41753, #48278 ) ;
#85779=DIRECTION ( 'NONE',  ( -1.000000000000000000, 6.938893903907222067E-15, 0.000000000000000000 ) ) ;
#85801=ADVANCED_FACE ( 'NONE', ( #74718, #66727, #50228 ), #21736, .T. ) ;
#85814=FACE_OUTER_BOUND ( 'NONE', #56410, .T. ) ;
#85851=AXIS2_PLACEMENT_3D ( 'NONE', #48825, #24508, #31481 ) ;
#85906=LINE ( 'NONE', #17420, #95201 ) ;
#85995=ORIENTED_EDGE ( 'NONE', *, *, #61925, .T. ) ;
#86007=DIRECTION ( 'NONE',  ( 1.000000000000000000, 0.000000000000000000, 0.000000000000000000 ) ) ;
#86057=CARTESIAN_POINT ( 'NONE',  ( 24.35999999999999233, 44.99999999999997158, 10.00000000000000000 ) ) ;
#86122=EDGE_CURVE ( 'NONE', #45903, #56516, #56766, .T. ) ;
#86134=DIRECTION ( 'NONE',  ( 0.1736481776669283605, -0.9848077530122084644, 0.000000000000000000 ) ) ;
#86165=ORIENTED_EDGE ( 'NONE', *, *, #75674, .F. ) ;
#86191=DIRECTION ( 'NONE',  ( -1.000000000000000000, 0.000000000000000000, 0.000000000000000000 ) ) ;
#86202=DIRECTION ( 'NONE',  ( -0.000000000000000000, -0.000000000000000000, -1.000000000000000000 ) ) ;
#86222=CARTESIAN_POINT ( 'NONE',  ( 34.56412365047464874, 29.50000000000000000, 9.500000000000000000 ) ) ;
#86257=DIRECTION ( 'NONE',  ( -5.818595309480553908E-17, -1.000000000000000000, -0.000000000000000000 ) ) ;
#86272=AXIS2_PLACEMENT_3D ( 'NONE', #72903, #78937, #11919 ) ;
#86305=DIRECTION ( 'NONE',  ( -1.000000000000000000, 0.000000000000000000, 0.000000000000000000 ) ) ;
#86330=CARTESIAN_POINT ( 'NONE',  ( 70.68973184038034674, 41.77083333333331439, -9.500000000000000000 ) ) ;
#86351=CIRCLE ( 'NONE', #84700, 19.99999999999999645 ) ;
#86365=LINE ( 'NONE', #88815, #14193 ) ;
#86386=EDGE_CURVE ( 'NONE', #1778, #1194, #87103, .T. ) ;
#86433=CARTESIAN_POINT ( 'NONE',  ( 26.00000000000000355, 35.99999999999997158, 7.000000000000000888 ) ) ;
#86451=CARTESIAN_POINT ( 'NONE',  ( 32.06412365047463453, 26.99999999999998224, 9.500000000000000000 ) ) ;
#86516=ORIENTED_EDGE ( 'NONE', *, *, #54745, .T. ) ;
#86525=DIRECTION ( 'NONE',  ( 0.000000000000000000, 0.000000000000000000, 1.000000000000000000 ) ) ;
#86570=LINE ( 'NONE', #56556, #62163 ) ;
#86581=ORIENTED_EDGE ( 'NONE', *, *, #68078, .F. ) ;
#86604=DIRECTION ( 'NONE',  ( -0.000000000000000000, -0.000000000000000000, -1.000000000000000000 ) ) ;
#86637=LINE ( 'NONE', #18146, #88857 ) ;
#86713=EDGE_LOOP ( 'NONE', ( #79967, #14607, #58579, #83892 ) ) ;
#86736=ORIENTED_EDGE ( 'NONE', *, *, #51145, .F. ) ;
#86750=VERTEX_POINT ( 'NONE', #60298 ) ;
#86892=AXIS2_PLACEMENT_3D ( 'NONE', #79013, #87007, #56032 ) ;
#86937=AXIS2_PLACEMENT_3D ( 'NONE', #18342, #48821, #38885 ) ;
#87006=EDGE_LOOP ( 'NONE', ( #10146, #40337, #38957, #31033 ) ) ;
#87007=DIRECTION ( 'NONE',  ( -0.000000000000000000, -0.000000000000000000, -1.000000000000000000 ) ) ;
#87042=DIRECTION ( 'NONE',  ( -1.000000000000000000, 0.000000000000000000, 0.000000000000000000 ) ) ;
#87103=CIRCLE ( 'NONE', #34418, 0.5000000000000000000 ) ;
#87112=SURFACE_STYLE_USAGE ( .BOTH. , #42606 ) ;
#87135=CIRCLE ( 'NONE', #86937, 0.4999999999999995559 ) ;
#87236=FACE_OUTER_BOUND ( 'NONE', #37780, .T. ) ;
#87256=CIRCLE ( 'NONE', #55367, 2.000000000000001776 ) ;
#87275=AXIS2_PLACEMENT_3D ( 'NONE', #72661, #81159, #89156 ) ;
#87279=VERTEX_POINT ( 'NONE', #68200 ) ;
#87393=CIRCLE ( 'NONE', #39528, 0.5000000000000004441 ) ;
#87399=VERTEX_POINT ( 'NONE', #78647 ) ;
#87416=DIRECTION ( 'NONE',  ( -0.000000000000000000, -0.000000000000000000, -1.000000000000000000 ) ) ;
#87419=DIRECTION ( 'NONE',  ( 0.000000000000000000, 1.000000000000000000, 0.000000000000000000 ) ) ;
#87445=VECTOR ( 'NONE', #90707, 1000.000000000000000 ) ;
#87478=CIRCLE ( 'NONE', #1301, 3.500000000000003109 ) ;
#87546=DIRECTION ( 'NONE',  ( -1.000000000000000000, 0.000000000000000000, 0.000000000000000000 ) ) ;
#87607=ORIENTED_EDGE ( 'NONE', *, *, #77894, .T. ) ;
#87730=ADVANCED_FACE ( 'NONE', ( #42608 ), #76113, .T. ) ;
#87737=FACE_OUTER_BOUND ( 'NONE', #19336, .T. ) ;
#87895=CIRCLE ( 'NONE', #86272, 0.5000000000000004441 ) ;
#87901=LINE ( 'NONE', #57409, #61170 ) ;
#87911=DIRECTION ( 'NONE',  ( 1.000000000000000000, 1.636349903325072848E-16, -0.000000000000000000 ) ) ;
#87942=AXIS2_PLACEMENT_3D ( 'NONE', #60204, #7217, #91696 ) ;
#87964=AXIS2_PLACEMENT_3D ( 'NONE', #19540, #97047, #59014 ) ;
#88014=DIRECTION ( 'NONE',  ( -0.9943711317468825195, -0.1059530667249610481, 0.000000000000000000 ) ) ;
#88053=AXIS2_PLACEMENT_3D ( 'NONE', #81648, #43166, #90629 ) ;
#88141=ADVANCED_FACE ( 'NONE', ( #32267 ), #49251, .T. ) ;
#88195=ORIENTED_EDGE ( 'NONE', *, *, #68784, .T. ) ;
#88213=DIRECTION ( 'NONE',  ( -0.000000000000000000, -0.000000000000000000, 1.000000000000000000 ) ) ;
#88290=DIRECTION ( 'NONE',  ( 0.1927083333333330095, -0.9812560818990572198, 0.000000000000000000 ) ) ;
#88394=EDGE_CURVE ( 'NONE', #48000, #56218, #33064, .T. ) ;
#88439=ORIENTED_EDGE ( 'NONE', *, *, #90792, .F. ) ;
#88477=DIRECTION ( 'NONE',  ( 1.000000000000000000, 0.000000000000000000, 0.000000000000000000 ) ) ;
#88503=CARTESIAN_POINT ( 'NONE',  ( -27.43587634952537968, 22.49999999999998934, -9.500000000000000000 ) ) ;
#88509=ORIENTED_EDGE ( 'NONE', *, *, #49890, .F. ) ;
#88552=ORIENTED_EDGE ( 'NONE', *, *, #20098, .T. ) ;
#88559=FACE_OUTER_BOUND ( 'NONE', #56240, .T. ) ;
#88592=ORIENTED_EDGE ( 'NONE', *, *, #11238, .F. ) ;
#88597=DIRECTION ( 'NONE',  ( 6.938893903907221278E-15, -1.000000000000000000, 0.000000000000000000 ) ) ;
#88602=ORIENTED_EDGE ( 'NONE', *, *, #56558, .F. ) ;
#88613=EDGE_CURVE ( 'NONE', #28657, #6038, #39441, .T. ) ;
#88644=CARTESIAN_POINT ( 'NONE',  ( 17.35999999999999943, 37.99999999999997868, 7.000000000000000000 ) ) ;
#88664=ORIENTED_EDGE ( 'NONE', *, *, #64320, .F. ) ;
#88711=AXIS2_PLACEMENT_3D ( 'NONE', #24722, #18199, #25709 ) ;
#88718=CARTESIAN_POINT ( 'NONE',  ( 24.35999999999999233, 44.99999999999999289, -7.000000000000000000 ) ) ;
#88782=DIRECTION ( 'NONE',  ( 0.9812560818990571088, 0.1927083333333329818, 0.000000000000000000 ) ) ;
#88788=VECTOR ( 'NONE', #96636, 1000.000000000000000 ) ;
#88815=CARTESIAN_POINT ( 'NONE',  ( 64.56412365047461321, 44.99999999999998579, 7.000000000000000000 ) ) ;
#88857=VECTOR ( 'NONE', #54155, 1000.000000000000000 ) ;
#88883=CIRCLE ( 'NONE', #17033, 19.99999999999999645 ) ;
#88884=CARTESIAN_POINT ( 'NONE',  ( 67.06412365047464164, 22.49999999999998934, -10.00000000000000000 ) ) ;
#88913=CIRCLE ( 'NONE', #45809, 1.499999999999996669 ) ;
#88959=DIRECTION ( 'NONE',  ( 1.000000000000000000, 0.000000000000000000, 0.000000000000000000 ) ) ;
#88976=CARTESIAN_POINT ( 'NONE',  ( 17.35999999999999943, 37.99999999999997868, 7.000000000000000000 ) ) ;
#89049=VERTEX_POINT ( 'NONE', #24189 ) ;
#89055=DIRECTION ( 'NONE',  ( -0.000000000000000000, -0.000000000000000000, -1.000000000000000000 ) ) ;
#89156=DIRECTION ( 'NONE',  ( 0.000000000000000000, 1.000000000000000000, 0.000000000000000000 ) ) ;
#89283=EDGE_CURVE ( 'NONE', #15070, #26787, #29849, .T. ) ;
#89286=ORIENTED_EDGE ( 'NONE', *, *, #20028, .F. ) ;
#89375=FACE_OUTER_BOUND ( 'NONE', #44375, .T. ) ;
#89581=AXIS2_PLACEMENT_3D ( 'NONE', #93801, #40814, #62309 ) ;
#89583=CARTESIAN_POINT ( 'NONE',  ( 24.35999999999999233, 44.99999999999999289, 7.000000000000000000 ) ) ;
#89590=CARTESIAN_POINT ( 'NONE',  ( -2.614810775378867191, 35.00346125376525919, 10.00000000000000000 ) ) ;
#89628=CARTESIAN_POINT ( 'NONE',  ( -2.283843307429720415, 13.12729635533385597, 9.500000000000000000 ) ) ;
#89639=ORIENTED_EDGE ( 'NONE', *, *, #25653, .F. ) ;
#89705=FACE_OUTER_BOUND ( 'NONE', #40202, .T. ) ;
#89737=CARTESIAN_POINT ( 'NONE',  ( 69.60148758828984228, 0.4999999999999982792, 10.00000000000000000 ) ) ;
#89841=DIRECTION ( 'NONE',  ( -0.000000000000000000, -0.000000000000000000, -1.000000000000000000 ) ) ;
#89859=DIRECTION ( 'NONE',  ( 1.000000000000000000, 0.000000000000000000, 0.000000000000000000 ) ) ;
#89887=DIRECTION ( 'NONE',  ( -0.000000000000000000, -0.000000000000000000, -1.000000000000000000 ) ) ;
#89936=AXIS2_PLACEMENT_3D ( 'NONE', #3186, #55693, #86191 ) ;
#89938=CARTESIAN_POINT ( 'NONE',  ( 69.60148758828984228, 0.4999999999999960032, 9.500000000000000000 ) ) ;
#89939=ORIENTED_EDGE ( 'NONE', *, *, #94315, .T. ) ;
#90049=ORIENTED_EDGE ( 'NONE', *, *, #8280, .F. ) ;
#90095=CIRCLE ( 'NONE', #86892, 1.999999999999996669 ) ;
#90181=CARTESIAN_POINT ( 'NONE',  ( -0.2838433074297238012, 13.12729635533385597, -9.500000000000000000 ) ) ;
#90195=LINE ( 'NONE', #44699, #2071 ) ;
#90415=CIRCLE ( 'NONE', #72850, 0.5000000000000004441 ) ;
#90537=EDGE_LOOP ( 'NONE', ( #65188, #3528, #86165, #22436 ) ) ;
#90546=CIRCLE ( 'NONE', #25048, 0.5000000000000000000 ) ;
#90608=DIRECTION ( 'NONE',  ( -1.000000000000000000, 0.000000000000000000, 0.000000000000000000 ) ) ;
#90629=DIRECTION ( 'NONE',  ( -1.000000000000000000, 5.818595309480552676E-17, 0.000000000000000000 ) ) ;
#90653=DIRECTION ( 'NONE',  ( -5.818595309480553908E-17, -1.000000000000000000, -0.000000000000000000 ) ) ;
#90681=VECTOR ( 'NONE', #17330, 1000.000000000000000 ) ;
#90707=DIRECTION ( 'NONE',  ( -0.000000000000000000, -0.000000000000000000, -1.000000000000000000 ) ) ;
#90717=CARTESIAN_POINT ( 'NONE',  ( 27.50000000000000355, 35.99999999999997158, -10.00000000000000000 ) ) ;
#90773=CARTESIAN_POINT ( 'NONE',  ( 17.85999999999999588, 33.98752635800203592, 10.00000000000000000 ) ) ;
#90781=ORIENTED_EDGE ( 'NONE', *, *, #82204, .F. ) ;
#90792=EDGE_CURVE ( 'NONE', #37315, #35951, #53066, .T. ) ;
#90824=( NAMED_UNIT ( * ) SI_UNIT ( $, .STERADIAN. ) SOLID_ANGLE_UNIT ( ) );
#90832=DIRECTION ( 'NONE',  ( 1.000000000000000000, 0.000000000000000000, -0.000000000000000000 ) ) ;
#90864=DIRECTION ( 'NONE',  ( 0.000000000000000000, 0.000000000000000000, -1.000000000000000000 ) ) ;
#90908=EDGE_CURVE ( 'NONE', #45908, #3546, #78607, .T. ) ;
#90936=EDGE_LOOP ( 'NONE', ( #97044, #28316, #40542, #78639 ) ) ;
#90969=CARTESIAN_POINT ( 'NONE',  ( 24.35999999999999233, 37.99999999999997868, 7.000000000000000000 ) ) ;
#90996=ORIENTED_EDGE ( 'NONE', *, *, #38299, .T. ) ;
#91196=EDGE_CURVE ( 'NONE', #46169, #35060, #5073, .T. ) ;
#91209=DIRECTION ( 'NONE',  ( -0.000000000000000000, -0.000000000000000000, -1.000000000000000000 ) ) ;
#91223=ORIENTED_EDGE ( 'NONE', *, *, #20344, .T. ) ;
#91264=CARTESIAN_POINT ( 'NONE',  ( 17.35999999999999588, 33.99999999999997868, 9.632054252037205444 ) ) ;
#91363=FACE_OUTER_BOUND ( 'NONE', #49284, .T. ) ;
#91378=DIRECTION ( 'NONE',  ( 0.000000000000000000, 0.000000000000000000, 1.000000000000000000 ) ) ;
#91409=AXIS2_PLACEMENT_3D ( 'NONE', #58369, #51880, #5407 ) ;
#91607=DIRECTION ( 'NONE',  ( 1.000000000000000000, 0.000000000000000000, 0.000000000000000000 ) ) ;
#91631=CARTESIAN_POINT ( 'NONE',  ( -2.614810775378867191, 35.00346125376525919, 7.000000000000000000 ) ) ;
#91633=ORIENTED_EDGE ( 'NONE', *, *, #46181, .F. ) ;
#91680=CARTESIAN_POINT ( 'NONE',  ( 34.56412365047463453, 26.99999999999999645, -9.500000000000000000 ) ) ;
#91692=DIRECTION ( 'NONE',  ( -1.000000000000000000, 0.000000000000000000, 0.000000000000000000 ) ) ;
#91696=DIRECTION ( 'NONE',  ( -1.000000000000000000, 0.000000000000000000, 0.000000000000000000 ) ) ;
#91778=ADVANCED_FACE ( 'NONE', ( #32976 ), #93984, .T. ) ;
#91842=FACE_OUTER_BOUND ( 'NONE', #72512, .T. ) ;
#91845=PLANE ( 'NONE',  #78378 ) ;
#91847=CIRCLE ( 'NONE', #75924, 1.499999999999996669 ) ;
#91930=CARTESIAN_POINT ( 'NONE',  ( 67.06412365047464164, 22.49999999999998934, -9.500000000000000000 ) ) ;
#92039=ORIENTED_EDGE ( 'NONE', *, *, #4170, .T. ) ;
#92054=AXIS2_PLACEMENT_3D ( 'NONE', #63641, #56169, #25675 ) ;
#92057=VERTEX_POINT ( 'NONE', #15916 ) ;
#92095=CARTESIAN_POINT ( 'NONE',  ( 56.78206182523731371, -3.303428494291771322E-15, 0.000000000000000000 ) ) ;
#92110=CARTESIAN_POINT ( 'NONE',  ( 31.00000000000000355, 44.99999999999999289, 7.000000000000000000 ) ) ;
#92126=ORIENTED_EDGE ( 'NONE', *, *, #14925, .T. ) ;
#92198=ORIENTED_EDGE ( 'NONE', *, *, #82319, .T. ) ;
#92206=ADVANCED_FACE ( 'NONE', ( #25878 ), #40399, .F. ) ;
#92229=VERTEX_POINT ( 'NONE', #93377 ) ;
#92271=AXIS2_PLACEMENT_3D ( 'NONE', #21012, #83481, #20516 ) ;
#92279=EDGE_CURVE ( 'NONE', #15047, #25147, #65873, .T. ) ;
#92308=( LENGTH_UNIT ( ) NAMED_UNIT ( * ) SI_UNIT ( .MILLI., .METRE. ) );
#92350=DIRECTION ( 'NONE',  ( -1.000000000000000000, 0.000000000000000000, 0.000000000000000000 ) ) ;
#92359=ADVANCED_FACE ( 'NONE', ( #27877 ), #59852, .T. ) ;
#92383=CARTESIAN_POINT ( 'NONE',  ( 69.60148758828984228, 0.4999999999999958922, -9.500000000000000000 ) ) ;
#92407=DIRECTION ( 'NONE',  ( -0.000000000000000000, -0.000000000000000000, -1.000000000000000000 ) ) ;
#92408=VECTOR ( 'NONE', #43704, 1000.000000000000000 ) ;
#92448=DIRECTION ( 'NONE',  ( 0.000000000000000000, -1.000000000000000000, 0.000000000000000000 ) ) ;
#92462=DIRECTION ( 'NONE',  ( 0.1736481776669282773, -0.9848077530122084644, 0.000000000000000000 ) ) ;
#92476=ORIENTED_EDGE ( 'NONE', *, *, #41817, .F. ) ;
#92486=ORIENTED_EDGE ( 'NONE', *, *, #54653, .F. ) ;
#92535=EDGE_LOOP ( 'NONE', ( #4935, #6310, #60921, #70829 ) ) ;
#92543=CARTESIAN_POINT ( 'NONE',  ( 66.76470751278411342, 44.99999999999998579, 9.500000000000000000 ) ) ;
#92622=VECTOR ( 'NONE', #50788, 1000.000000000000000 ) ;
#92633=AXIS2_PLACEMENT_3D ( 'NONE', #37416, #91378, #97931 ) ;
#92677=EDGE_LOOP ( 'NONE', ( #50094, #34844, #20900, #78618 ) ) ;
#92731=AXIS2_PLACEMENT_3D ( 'NONE', #75088, #45580, #83086 ) ;
#92758=ORIENTED_EDGE ( 'NONE', *, *, #86122, .T. ) ;
#92788=AXIS2_PLACEMENT_3D ( 'NONE', #9322, #85320, #56307 ) ;
#92821=DIRECTION ( 'NONE',  ( -1.000000000000000000, -0.000000000000000000, -0.000000000000000000 ) ) ;
#92910=EDGE_CURVE ( 'NONE', #6038, #26787, #77084, .T. ) ;
#93091=CARTESIAN_POINT ( 'NONE',  ( 64.56412365047462742, 13.99999999999999467, 9.500000000000000000 ) ) ;
#93139=CIRCLE ( 'NONE', #38843, 0.5000000000000004441 ) ;
#93142=CIRCLE ( 'NONE', #97967, 0.5000000000000004441 ) ;
#93248=ADVANCED_FACE ( 'NONE', ( #63932 ), #84501, .F. ) ;
#93263=VERTEX_POINT ( 'NONE', #16001 ) ;
#93264=ORIENTED_EDGE ( 'NONE', *, *, #8493, .T. ) ;
#93308=FACE_OUTER_BOUND ( 'NONE', #1435, .T. ) ;
#93377=CARTESIAN_POINT ( 'NONE',  ( 38.04706783004212411, -5.848780422071338384E-15, 7.000000000000000000 ) ) ;
#93438=CARTESIAN_POINT ( 'NONE',  ( 70.08911253270098030, 0.3894472361808988259, 9.500000000000000000 ) ) ;
#93453=CARTESIAN_POINT ( 'NONE',  ( -1.761054936948033056, 12.86682408883346440, -9.500000000000000000 ) ) ;
#93462=AXIS2_PLACEMENT_3D ( 'NONE', #40292, #2318, #93776 ) ;
#93515=ORIENTED_EDGE ( 'NONE', *, *, #62975, .T. ) ;
#93527=DIRECTION ( 'NONE',  ( 1.000000000000000000, 1.636349903325072848E-16, -0.000000000000000000 ) ) ;
#93591=CIRCLE ( 'NONE', #50481, 0.5000000000000066613 ) ;
#93593=ORIENTED_EDGE ( 'NONE', *, *, #4446, .T. ) ;
#93705=CARTESIAN_POINT ( 'NONE',  ( 27.50000000000000355, 35.99999999999997158, 10.00000000000000000 ) ) ;
#93722=AXIS2_PLACEMENT_3D ( 'NONE', #8024, #25496, #46988 ) ;
#93739=EDGE_LOOP ( 'NONE', ( #88195, #82911, #32848, #40974 ) ) ;
#93776=DIRECTION ( 'NONE',  ( -1.000000000000000000, 0.000000000000000000, 0.000000000000000000 ) ) ;
#93801=CARTESIAN_POINT ( 'NONE',  ( 34.56412365047463453, 13.99999999999999645, 9.500000000000000000 ) ) ;
#93805=ADVANCED_FACE ( 'NONE', ( #68961 ), #84457, .T. ) ;
#93884=VECTOR ( 'NONE', #51100, 1000.000000000000000 ) ;
#93984=PLANE ( 'NONE',  #3627 ) ;
#94079=DIRECTION ( 'NONE',  ( -0.000000000000000000, -0.000000000000000000, -1.000000000000000000 ) ) ;
#94095=PLANE ( 'NONE',  #28354 ) ;
#94111=CARTESIAN_POINT ( 'NONE',  ( 24.35999999999999233, 37.99999999999997868, 10.00000000000000000 ) ) ;
#94231=ORIENTED_EDGE ( 'NONE', *, *, #7735, .F. ) ;
#94256=CARTESIAN_POINT ( 'NONE',  ( 38.04706783004212411, 44.99999999999999289, 7.000000000000000000 ) ) ;
#94279=DIRECTION ( 'NONE',  ( 1.000000000000000000, -5.782411586589362323E-17, 0.000000000000000000 ) ) ;
#94289=VERTEX_POINT ( 'NONE', #90717 ) ;
#94314=AXIS2_PLACEMENT_3D ( 'NONE', #56754, #56279, #73225 ) ;
#94315=EDGE_CURVE ( 'NONE', #20515, #87279, #21391, .T. ) ;
#94367=EDGE_CURVE ( 'NONE', #84180, #38557, #31016, .T. ) ;
#94387=EDGE_CURVE ( 'NONE', #63343, #57472, #7056, .T. ) ;
#94409=DIRECTION ( 'NONE',  ( -1.000000000000000000, 0.000000000000000000, 0.000000000000000000 ) ) ;
#94413=ORIENTED_EDGE ( 'NONE', *, *, #22911, .F. ) ;
#94425=CYLINDRICAL_SURFACE ( 'NONE', #60645, 0.5000000000000004441 ) ;
#94630=CIRCLE ( 'NONE', #75440, 2.500000000000002220 ) ;
#94646=EDGE_CURVE ( 'NONE', #57472, #295, #23051, .T. ) ;
#94696=LINE ( 'NONE', #9723, #2602 ) ;
#94743=ADVANCED_FACE ( 'NONE', ( #19154 ), #26646, .T. ) ;
#94778=CARTESIAN_POINT ( 'NONE',  ( 66.56412365047464164, 26.99999999999998224, 10.00000000000000000 ) ) ;
#94846=VERTEX_POINT ( 'NONE', #11650 ) ;
#94853=CARTESIAN_POINT ( 'NONE',  ( 24.35999999999999233, 37.99999999999997868, 9.500000000000000000 ) ) ;
#94980=ORIENTED_EDGE ( 'NONE', *, *, #63217, .F. ) ;
#94996=ORIENTED_EDGE ( 'NONE', *, *, #34653, .T. ) ;
#95088=VECTOR ( 'NONE', #75457, 1000.000000000000000 ) ;
#95101=EDGE_CURVE ( 'NONE', #44442, #50694, #30090, .T. ) ;
#95118=CYLINDRICAL_SURFACE ( 'NONE', #41644, 0.5000000000000000000 ) ;
#95201=VECTOR ( 'NONE', #77397, 1000.000000000000000 ) ;
#95355=ORIENTED_EDGE ( 'NONE', *, *, #63270, .F. ) ;
#95361=CARTESIAN_POINT ( 'NONE',  ( -0.4427729075171641382, 14.61885305295417048, 10.00000000000000000 ) ) ;
#95570=DIRECTION ( 'NONE',  ( 0.9848077530122084644, 0.1736481776669281663, 0.000000000000000000 ) ) ;
#95577=DIRECTION ( 'NONE',  ( -1.000000000000000000, 0.000000000000000000, 0.000000000000000000 ) ) ;
#95591=EDGE_LOOP ( 'NONE', ( #805, #83293 ) ) ;
#95638=ORIENTED_EDGE ( 'NONE', *, *, #51915, .T. ) ;
#95647=DIRECTION ( 'NONE',  ( 0.000000000000000000, 0.000000000000000000, 1.000000000000000000 ) ) ;
#95715=DIRECTION ( 'NONE',  ( 0.000000000000000000, 0.000000000000000000, -1.000000000000000000 ) ) ;
#95774=TOROIDAL_SURFACE ( 'NONE', #73418, 6.499999999999995559, 0.5000000000000000000 ) ;
#95843=ORIENTED_EDGE ( 'NONE', *, *, #59434, .T. ) ;
#95852=CARTESIAN_POINT ( 'NONE',  ( 5.000000000000002665, 44.99999999999999289, 7.000000000000000000 ) ) ;
#95909=ORIENTED_EDGE ( 'NONE', *, *, #34474, .F. ) ;
#96026=ORIENTED_EDGE ( 'NONE', *, *, #5462, .F. ) ;
#96118=FACE_OUTER_BOUND ( 'NONE', #66153, .T. ) ;
#96124=CARTESIAN_POINT ( 'NONE',  ( 32.06412365047463453, 26.99999999999997868, 9.500000000000000000 ) ) ;
#96156=CYLINDRICAL_SURFACE ( 'NONE', #62741, 2.000000000000001776 ) ;
#96214=AXIS2_PLACEMENT_3D ( 'NONE', #80678, #72183, #65166 ) ;
#96225=VECTOR ( 'NONE', #14467, 1000.000000000000000 ) ;
#96231=CARTESIAN_POINT ( 'NONE',  ( 26.00000000000000355, 35.99999999999997158, -10.00000000000000000 ) ) ;
#96262=AXIS2_PLACEMENT_3D ( 'NONE', #71756, #3266, #18767 ) ;
#96265=DIRECTION ( 'NONE',  ( -1.000000000000000000, 0.000000000000000000, 0.000000000000000000 ) ) ;
#96396=ORIENTED_EDGE ( 'NONE', *, *, #45490, .T. ) ;
#96493=DIRECTION ( 'NONE',  ( 0.000000000000000000, 1.000000000000000000, -6.938893903907221278E-15 ) ) ;
#96502=DIRECTION ( 'NONE',  ( 0.9848077530122086864, 0.1736481776669271671, 0.000000000000000000 ) ) ;
#96569=DIRECTION ( 'NONE',  ( 0.1736481776669272503, -0.9848077530122086864, 0.000000000000000000 ) ) ;
#96613=( GEOMETRIC_REPRESENTATION_CONTEXT ( 3 ) GLOBAL_UNCERTAINTY_ASSIGNED_CONTEXT ( ( #82465 ) ) GLOBAL_UNIT_ASSIGNED_CONTEXT ( ( #45837, #363, #90824 ) ) REPRESENTATION_CONTEXT ( 'NONE', 'WORKASPACE' ) );
#96629=LINE ( 'NONE', #22105, #45131 ) ;
#96636=DIRECTION ( 'NONE',  ( -0.000000000000000000, -0.000000000000000000, -1.000000000000000000 ) ) ;
#96792=ORIENTED_EDGE ( 'NONE', *, *, #65690, .F. ) ;
#96810=ORIENTED_EDGE ( 'NONE', *, *, #7017, .F. ) ;
#96886=TOROIDAL_SURFACE ( 'NONE', #93722, 2.500000000000001776, 0.5000000000000000000 ) ;
#96917=DIRECTION ( 'NONE',  ( -5.818595309480553908E-17, -1.000000000000000000, -0.000000000000000000 ) ) ;
#96926=CARTESIAN_POINT ( 'NONE',  ( 64.56412365047461321, 29.50000000000000000, 10.00000000000000000 ) ) ;
#96929=DIRECTION ( 'NONE',  ( -0.000000000000000000, -0.000000000000000000, -1.000000000000000000 ) ) ;
#97002=ADVANCED_FACE ( 'NONE', ( #24257 ), #40230, .T. ) ;
#97044=ORIENTED_EDGE ( 'NONE', *, *, #82204, .T. ) ;
#97047=DIRECTION ( 'NONE',  ( 1.000000000000000000, -8.673617379884027583E-16, 0.000000000000000000 ) ) ;
#97091=ORIENTED_EDGE ( 'NONE', *, *, #71268, .T. ) ;
#97151=EDGE_CURVE ( 'NONE', #45908, #18967, #646, .T. ) ;
#97209=ORIENTED_EDGE ( 'NONE', *, *, #38954, .F. ) ;
#97352=CIRCLE ( 'NONE', #1577, 0.5000000000000000000 ) ;
#97387=CARTESIAN_POINT ( 'NONE',  ( 69.60148758828984228, 0.4999999999999982792, 9.500000000000000000 ) ) ;
#97497=CIRCLE ( 'NONE', #49570, 20.49999999999999645 ) ;
#97501=CARTESIAN_POINT ( 'NONE',  ( 2.618367889266248100E-15, 44.99999999999999289, 7.000000000000000000 ) ) ;
#97507=AXIS2_PLACEMENT_3D ( 'NONE', #73833, #74318, #58327 ) ;
#97546=EDGE_CURVE ( 'NONE', #62023, #41634, #67706, .T. ) ;
#97547=DIRECTION ( 'NONE',  ( 0.000000000000000000, 1.000000000000000000, -0.000000000000000000 ) ) ;
#97553=DIRECTION ( 'NONE',  ( 0.000000000000000000, 0.000000000000000000, 1.000000000000000000 ) ) ;
#97602=EDGE_LOOP ( 'NONE', ( #55909, #21123, #24146, #64470 ) ) ;
#97613=ORIENTED_EDGE ( 'NONE', *, *, #73553, .T. ) ;
#97623=CARTESIAN_POINT ( 'NONE',  ( 64.56412365047461321, 29.50000000000000000, 10.00000000000000000 ) ) ;
#97632=AXIS2_PLACEMENT_3D ( 'NONE', #12640, #66129, #97653 ) ;
#97633=ORIENTED_EDGE ( 'NONE', *, *, #50729, .T. ) ;
#97649=AXIS2_PLACEMENT_3D ( 'NONE', #91631, #77109, #70608 ) ;
#97653=DIRECTION ( 'NONE',  ( 1.000000000000000000, 0.000000000000000000, 0.000000000000000000 ) ) ;
#97671=FACE_OUTER_BOUND ( 'NONE', #64584, .T. ) ;
#97730=ORIENTED_EDGE ( 'NONE', *, *, #90908, .F. ) ;
#97831=CIRCLE ( 'NONE', #14820, 0.5000000000000004441 ) ;
#97895=EDGE_LOOP ( 'NONE', ( #12972, #36521, #90049, #70684 ) ) ;
#97920=EDGE_CURVE ( 'NONE', #63150, #46169, #90095, .T. ) ;
#97931=DIRECTION ( 'NONE',  ( -1.000000000000000000, 2.081668171172166620E-14, 0.000000000000000000 ) ) ;
#97967=AXIS2_PLACEMENT_3D ( 'NONE', #65966, #96493, #27966 ) ;
#98033=CARTESIAN_POINT ( 'NONE',  ( 64.56412365047461321, 44.99999999999998579, -7.000000000000000000 ) ) ;
#98052=DIRECTION ( 'NONE',  ( 0.000000000000000000, 0.000000000000000000, -1.000000000000000000 ) ) ;
#98070=LINE ( 'NONE', #65557, #24298 ) ;
#98257=DIRECTION ( 'NONE',  ( 1.000000000000000000, -5.782411586589362323E-17, 0.000000000000000000 ) ) ;
#98260=CARTESIAN_POINT ( 'NONE',  ( 67.06412365047464164, 14.00000000000000888, -9.500000000000000000 ) ) ;
#98287=DIRECTION ( 'NONE',  ( -1.000000000000000000, 0.000000000000000000, 0.000000000000000000 ) ) ;
#98366=TOROIDAL_SURFACE ( 'NONE', #44007, 3.500000000000000888, 0.5000000000000000000 ) ;
#98382=LINE ( 'NONE', #29838, #63321 ) ;
#98426=CARTESIAN_POINT ( 'NONE',  ( 24.50000000000000000, 35.99999999999997158, -10.00000000000000000 ) ) ;
#98464=COLOUR_RGB ( '', 0.72549020, 0.75294118, 0.79215686) ;
#98492=LINE ( 'NONE', #5988, #95088 ) ;
#98533=DIRECTION ( 'NONE',  ( -0.9812560818990571088, -0.1927083333333329818, 0.000000000000000000 ) ) ;
#98544=DIRECTION ( 'NONE',  ( 5.818595309480553908E-17, 1.000000000000000000, 0.000000000000000000 ) ) ;
#98561=CARTESIAN_POINT ( 'NONE',  ( 17.35999999999999943, 33.99999999999997158, 9.500000000000000000 ) ) ;
#98573=AXIS2_PLACEMENT_3D ( 'NONE', #96124, #88597, #12604 ) ;
#98582=APPLICATION_CONTEXT ( 'automotive_design' ) ;
#98584=AXIS2_PLACEMENT_3D ( 'NONE', #86433, #64873, #2463 ) ;
#98661=CARTESIAN_POINT ( 'NONE',  ( -4.182615635448458491, 26.60017725333985794, 10.00000000000000000 ) ) ;
#98734=LINE ( 'NONE', #4873, #17194 ) ;
#98757=DIRECTION ( 'NONE',  ( 0.000000000000000000, 0.000000000000000000, 1.000000000000000000 ) ) ;
#98777=DIRECTION ( 'NONE',  ( -0.000000000000000000, -0.000000000000000000, -1.000000000000000000 ) ) ;
#98814=EDGE_LOOP ( 'NONE', ( #69887, #16253, #24878, #80601, #4639, #94996 ) ) ;
#98843=CARTESIAN_POINT ( 'NONE',  ( 69.60148758828984228, -4.049828892140921146E-15, -9.500000000000000000 ) ) ;
#98847=DIRECTION ( 'NONE',  ( -1.000000000000000000, 0.000000000000000000, 0.000000000000000000 ) ) ;
#98885=DIRECTION ( 'NONE',  ( 1.636349903325072848E-16, -1.000000000000000000, 0.000000000000000000 ) ) ;
ENDSEC;
END-ISO-10303-21;
